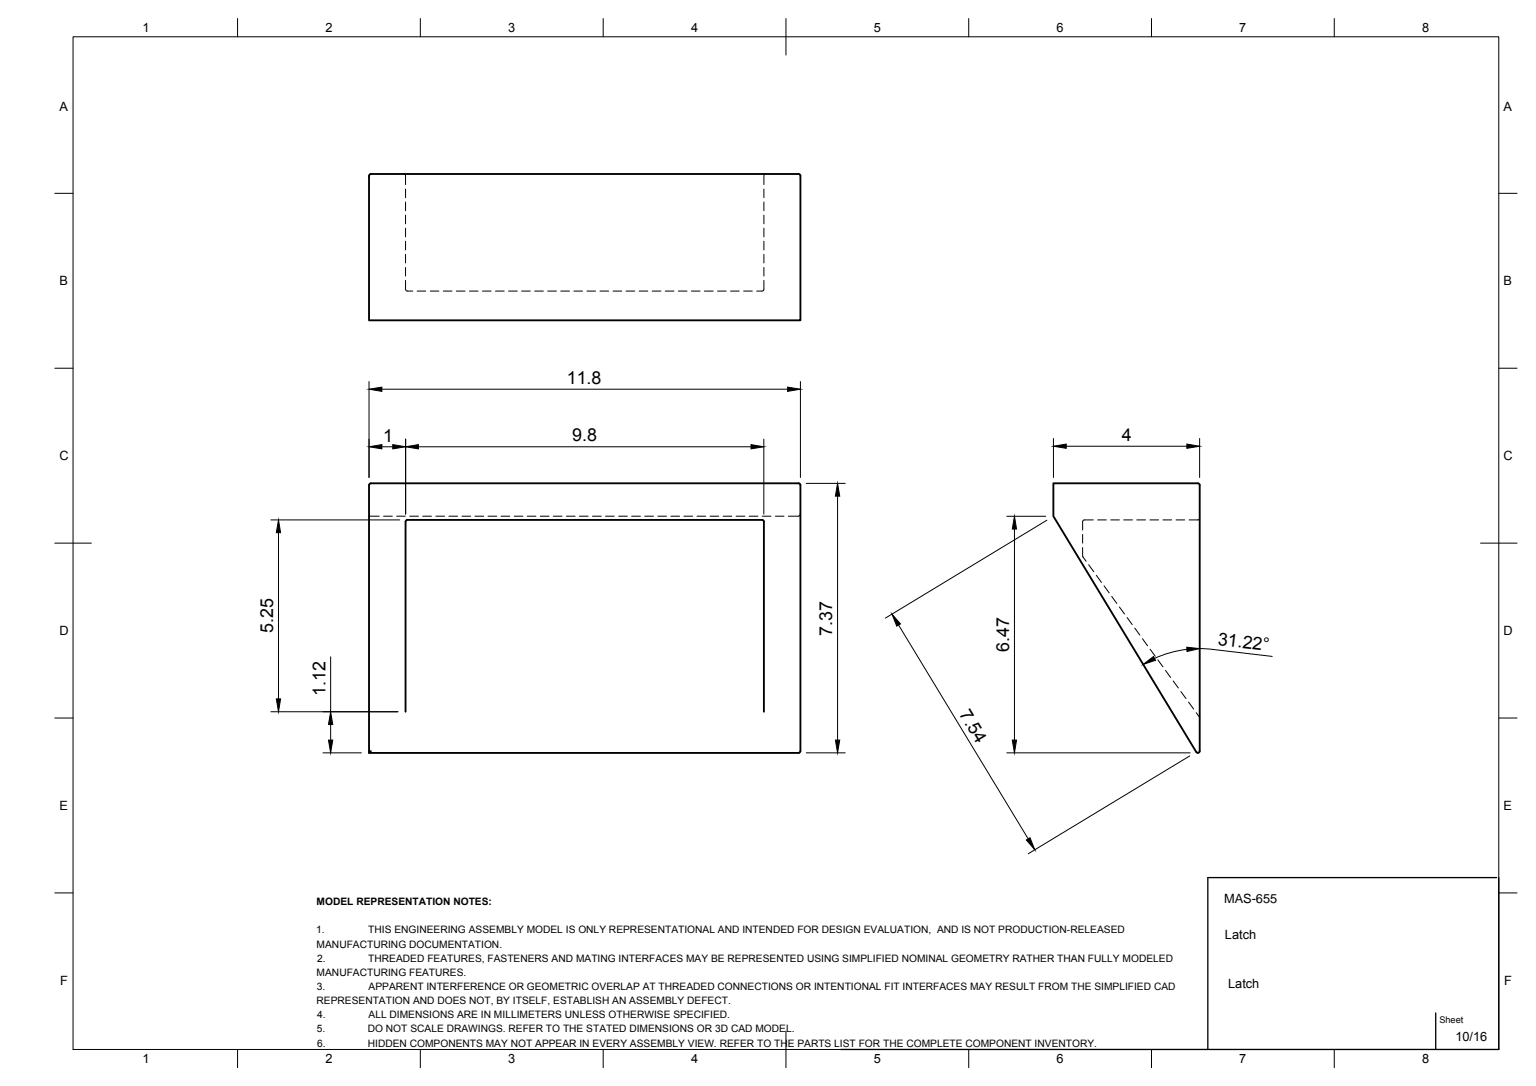
ISO-10303-21;
HEADER;
FILE_DESCRIPTION((''),'2;1');
FILE_NAME('Latch.step','2026-10-09T11:34:15-07:00',(''),(''),'','','');
FILE_SCHEMA (('AUTOMOTIVE_DESIGN { 1 0 10303 214 3 1 1 }'));
ENDSEC;
DATA;
#10=MECHANICAL_DESIGN_GEOMETRIC_PRESENTATION_REPRESENTATION('',(#642),#117170);
#389=ELLIPSE('',#52464,0.170018381359192,0.0999999999999989) ;
#390=ELLIPSE('',#52466,0.146308748884013,0.0499999999999989) ;
#391=ELLIPSE('',#52481,0.170018381359207,0.100000000000008) ;
#392=ELLIPSE('',#52483,0.146308748884017,0.0499999999999989) ;
#393=ELLIPSE('',#52506,0.0707106781186453,0.05) ;
#394=ELLIPSE('',#52515,0.0964689069078737,0.05) ;
#600=SHAPE_REPRESENTATION_RELATIONSHIP('SRR','None',#117255,#621) ;
#621=ADVANCED_BREP_SHAPE_REPRESENTATION('',(#663),#117163) ;
#642=STYLED_ITEM('',(#117355),#663) ;
#663=MANIFOLD_SOLID_BREP('Body1',#49071) ;
#737=FACE_BOUND('',#15539,.T.) ;
#2003=B_SPLINE_SURFACE_WITH_KNOTS('',3,3,((#88809,#88810,#88811,#88812,
#88813,#88814),(#88815,#88816,#88817,#88818,#88819,#88820),(#88821,#88822,
#88823,#88824,#88825,#88826),(#88827,#88828,#88829,#88830,#88831,#88832),
(#88833,#88834,#88835,#88836,#88837,#88838)),.UNSPECIFIED.,.F.,.F.,.F.,
(4,1,4),(4,1,1,4),(-0.00263861939634921,0.571428571428571,1.),(4.70975036097816,
5.38558740615393,5.83438635666676,6.28582392658612),.UNSPECIFIED.) ;
#2004=B_SPLINE_SURFACE_WITH_KNOTS('',3,3,((#88875,#88876,#88877,#88878,
#88879),(#88880,#88881,#88882,#88883,#88884),(#88885,#88886,#88887,#88888,
#88889),(#88890,#88891,#88892,#88893,#88894),(#88895,#88896,#88897,#88898,
#88899)),.UNSPECIFIED.,.F.,.F.,.F.,(4,1,4),(4,1,4),(-0.00515447126046521,
0.571428571428571,1.00290951547842),(-0.00515447124447774,0.673198425769152,
1.5759507980487),.UNSPECIFIED.) ;
#2204=SPHERICAL_SURFACE('',#52445,0.0499999999999989) ;
#2205=SPHERICAL_SURFACE('',#52449,0.0499999999999989) ;
#2206=SPHERICAL_SURFACE('',#52454,0.0499999999999901) ;
#2207=SPHERICAL_SURFACE('',#52470,0.0499999999999945) ;
#2208=SPHERICAL_SURFACE('',#52496,0.0499999999999989) ;
#2209=SPHERICAL_SURFACE('',#52500,0.0499999999999989) ;
#2210=SPHERICAL_SURFACE('',#52507,0.0499999999999989) ;
#2552=PLANE('',#52491) ;
#2553=PLANE('',#52492) ;
#2554=PLANE('',#52493) ;
#2555=PLANE('',#52494) ;
#2556=PLANE('',#52495) ;
#2557=PLANE('',#52520) ;
#2558=PLANE('',#52521) ;
#2559=PLANE('',#52522) ;
#2560=PLANE('',#52523) ;
#2561=PLANE('',#52524) ;
#2562=PLANE('',#52525) ;
#4549=LINE('',#88788,#7763) ;
#4550=LINE('',#88789,#7764) ;
#4551=LINE('',#88798,#7765) ;
#4552=LINE('',#88799,#7766) ;
#4553=LINE('',#88848,#7767) ;
#4554=LINE('',#88849,#7768) ;
#4555=LINE('',#88851,#7769) ;
#4556=LINE('',#88852,#7770) ;
#4557=LINE('',#88861,#7771) ;
#4558=LINE('',#88862,#7772) ;
#4559=LINE('',#88864,#7773) ;
#4560=LINE('',#88865,#7774) ;
#4561=LINE('',#88909,#7775) ;
#4562=LINE('',#88910,#7776) ;
#4563=LINE('',#88912,#7777) ;
#4564=LINE('',#88913,#7778) ;
#4565=LINE('',#88915,#7779) ;
#4566=LINE('',#88916,#7780) ;
#4567=LINE('',#88918,#7781) ;
#4568=LINE('',#88919,#7782) ;
#4569=LINE('',#88921,#7783) ;
#4570=LINE('',#88922,#7784) ;
#4571=LINE('',#88924,#7785) ;
#4572=LINE('',#88925,#7786) ;
#4573=LINE('',#88946,#7787) ;
#4574=LINE('',#88947,#7788) ;
#4575=LINE('',#88950,#7789) ;
#4576=LINE('',#88952,#7790) ;
#4577=LINE('',#88962,#7791) ;
#4578=LINE('',#88963,#7792) ;
#4579=LINE('',#88966,#7793) ;
#4580=LINE('',#88967,#7794) ;
#4581=LINE('',#88973,#7795) ;
#4582=LINE('',#88974,#7796) ;
#4583=LINE('',#88979,#7797) ;
#4584=LINE('',#88980,#7798) ;
#4585=LINE('',#88985,#7799) ;
#4586=LINE('',#88986,#7800) ;
#4587=LINE('',#88988,#7801) ;
#4588=LINE('',#88991,#7802) ;
#4589=LINE('',#88992,#7803) ;
#4590=LINE('',#88993,#7804) ;
#4591=LINE('',#88995,#7805) ;
#7763=VECTOR('',#62902,10.) ;
#7764=VECTOR('',#62903,10.) ;
#7765=VECTOR('',#62914,10.) ;
#7766=VECTOR('',#62915,10.) ;
#7767=VECTOR('',#62936,10.) ;
#7768=VECTOR('',#62937,10.) ;
#7769=VECTOR('',#62940,10.) ;
#7770=VECTOR('',#62941,10.) ;
#7771=VECTOR('',#62952,10.) ;
#7772=VECTOR('',#62953,10.) ;
#7773=VECTOR('',#62956,10.) ;
#7774=VECTOR('',#62957,10.) ;
#7775=VECTOR('',#62978,10.) ;
#7776=VECTOR('',#62979,10.) ;
#7777=VECTOR('',#62982,10.) ;
#7778=VECTOR('',#62983,10.) ;
#7779=VECTOR('',#62986,10.) ;
#7780=VECTOR('',#62987,10.) ;
#7781=VECTOR('',#62990,10.) ;
#7782=VECTOR('',#62991,10.) ;
#7783=VECTOR('',#62994,10.) ;
#7784=VECTOR('',#62995,10.) ;
#7785=VECTOR('',#62998,10.) ;
#7786=VECTOR('',#62999,10.) ;
#7787=VECTOR('',#63028,10.) ;
#7788=VECTOR('',#63029,10.) ;
#7789=VECTOR('',#63032,10.) ;
#7790=VECTOR('',#63033,10.) ;
#7791=VECTOR('',#63046,10.) ;
#7792=VECTOR('',#63047,10.) ;
#7793=VECTOR('',#63050,10.) ;
#7794=VECTOR('',#63051,10.) ;
#7795=VECTOR('',#63058,10.) ;
#7796=VECTOR('',#63059,10.) ;
#7797=VECTOR('',#63064,10.) ;
#7798=VECTOR('',#63065,10.) ;
#7799=VECTOR('',#63070,10.) ;
#7800=VECTOR('',#63071,10.) ;
#7801=VECTOR('',#63074,10.) ;
#7802=VECTOR('',#63077,10.) ;
#7803=VECTOR('',#63078,10.) ;
#7804=VECTOR('',#63079,10.) ;
#7805=VECTOR('',#63082,10.) ;
#10115=CYLINDRICAL_SURFACE('',#52453,0.05) ;
#10116=CYLINDRICAL_SURFACE('',#52458,0.05) ;
#10117=CYLINDRICAL_SURFACE('',#52468,0.05) ;
#10118=CYLINDRICAL_SURFACE('',#52469,0.05) ;
#10119=CYLINDRICAL_SURFACE('',#52474,0.05) ;
#10120=CYLINDRICAL_SURFACE('',#52475,0.05) ;
#10121=CYLINDRICAL_SURFACE('',#52485,0.05) ;
#10122=CYLINDRICAL_SURFACE('',#52486,0.05) ;
#10123=CYLINDRICAL_SURFACE('',#52487,0.05) ;
#10124=CYLINDRICAL_SURFACE('',#52488,0.05) ;
#10125=CYLINDRICAL_SURFACE('',#52489,0.05) ;
#10126=CYLINDRICAL_SURFACE('',#52490,0.05) ;
#10127=CYLINDRICAL_SURFACE('',#52504,0.05) ;
#10128=CYLINDRICAL_SURFACE('',#52505,0.05) ;
#10129=CYLINDRICAL_SURFACE('',#52511,0.05) ;
#10130=CYLINDRICAL_SURFACE('',#52512,0.05) ;
#10131=CYLINDRICAL_SURFACE('',#52514,0.05) ;
#10132=CYLINDRICAL_SURFACE('',#52516,0.05) ;
#10133=CYLINDRICAL_SURFACE('',#52518,0.05) ;
#12341=FACE_OUTER_BOUND('',#15500,.T.) ;
#12342=FACE_OUTER_BOUND('',#15501,.T.) ;
#12343=FACE_OUTER_BOUND('',#15502,.T.) ;
#12344=FACE_OUTER_BOUND('',#15503,.T.) ;
#12345=FACE_OUTER_BOUND('',#15504,.T.) ;
#12346=FACE_OUTER_BOUND('',#15505,.T.) ;
#12347=FACE_OUTER_BOUND('',#15506,.T.) ;
#12348=FACE_OUTER_BOUND('',#15507,.T.) ;
#12349=FACE_OUTER_BOUND('',#15508,.T.) ;
#12350=FACE_OUTER_BOUND('',#15509,.T.) ;
#12351=FACE_OUTER_BOUND('',#15510,.T.) ;
#12352=FACE_OUTER_BOUND('',#15511,.T.) ;
#12353=FACE_OUTER_BOUND('',#15512,.T.) ;
#12354=FACE_OUTER_BOUND('',#15513,.T.) ;
#12355=FACE_OUTER_BOUND('',#15514,.T.) ;
#12356=FACE_OUTER_BOUND('',#15515,.T.) ;
#12357=FACE_OUTER_BOUND('',#15516,.T.) ;
#12358=FACE_OUTER_BOUND('',#15517,.T.) ;
#12359=FACE_OUTER_BOUND('',#15518,.T.) ;
#12360=FACE_OUTER_BOUND('',#15519,.T.) ;
#12361=FACE_OUTER_BOUND('',#15520,.T.) ;
#12362=FACE_OUTER_BOUND('',#15521,.T.) ;
#12363=FACE_OUTER_BOUND('',#15522,.T.) ;
#12364=FACE_OUTER_BOUND('',#15523,.T.) ;
#12365=FACE_OUTER_BOUND('',#15524,.T.) ;
#12366=FACE_OUTER_BOUND('',#15525,.T.) ;
#12367=FACE_OUTER_BOUND('',#15526,.T.) ;
#12368=FACE_OUTER_BOUND('',#15527,.T.) ;
#12369=FACE_OUTER_BOUND('',#15528,.T.) ;
#12370=FACE_OUTER_BOUND('',#15529,.T.) ;
#12371=FACE_OUTER_BOUND('',#15530,.T.) ;
#12372=FACE_OUTER_BOUND('',#15531,.T.) ;
#12373=FACE_OUTER_BOUND('',#15532,.T.) ;
#12374=FACE_OUTER_BOUND('',#15533,.T.) ;
#12375=FACE_OUTER_BOUND('',#15534,.T.) ;
#12376=FACE_OUTER_BOUND('',#15535,.T.) ;
#12377=FACE_OUTER_BOUND('',#15536,.T.) ;
#12378=FACE_OUTER_BOUND('',#15537,.T.) ;
#12379=FACE_OUTER_BOUND('',#15538,.T.) ;
#12380=FACE_OUTER_BOUND('',#15540,.T.) ;
#12381=FACE_OUTER_BOUND('',#15541,.T.) ;
#15500=EDGE_LOOP('',(#38300,#38301,#38302)) ;
#15501=EDGE_LOOP('',(#38303,#38304,#38305)) ;
#15502=EDGE_LOOP('',(#38306,#38307,#38308,#38309)) ;
#15503=EDGE_LOOP('',(#38310,#38311,#38312)) ;
#15504=EDGE_LOOP('',(#38313,#38314,#38315,#38316)) ;
#15505=EDGE_LOOP('',(#38317,#38318,#38319,#38320)) ;
#15506=EDGE_LOOP('',(#38321,#38322,#38323,#38324)) ;
#15507=EDGE_LOOP('',(#38325,#38326,#38327,#38328)) ;
#15508=EDGE_LOOP('',(#38329,#38330,#38331,#38332)) ;
#15509=EDGE_LOOP('',(#38333,#38334,#38335)) ;
#15510=EDGE_LOOP('',(#38336,#38337,#38338,#38339)) ;
#15511=EDGE_LOOP('',(#38340,#38341,#38342,#38343)) ;
#15512=EDGE_LOOP('',(#38344,#38345,#38346,#38347)) ;
#15513=EDGE_LOOP('',(#38348,#38349,#38350,#38351)) ;
#15514=EDGE_LOOP('',(#38352,#38353,#38354,#38355)) ;
#15515=EDGE_LOOP('',(#38356,#38357,#38358,#38359)) ;
#15516=EDGE_LOOP('',(#38360,#38361,#38362,#38363)) ;
#15517=EDGE_LOOP('',(#38364,#38365,#38366,#38367)) ;
#15518=EDGE_LOOP('',(#38368,#38369,#38370,#38371)) ;
#15519=EDGE_LOOP('',(#38372,#38373,#38374,#38375)) ;
#15520=EDGE_LOOP('',(#38376,#38377,#38378,#38379)) ;
#15521=EDGE_LOOP('',(#38380,#38381,#38382,#38383)) ;
#15522=EDGE_LOOP('',(#38384,#38385,#38386,#38387)) ;
#15523=EDGE_LOOP('',(#38388,#38389,#38390,#38391)) ;
#15524=EDGE_LOOP('',(#38392,#38393,#38394,#38395)) ;
#15525=EDGE_LOOP('',(#38396,#38397,#38398)) ;
#15526=EDGE_LOOP('',(#38399,#38400,#38401)) ;
#15527=EDGE_LOOP('',(#38402,#38403,#38404,#38405)) ;
#15528=EDGE_LOOP('',(#38406,#38407,#38408,#38409)) ;
#15529=EDGE_LOOP('',(#38410,#38411,#38412)) ;
#15530=EDGE_LOOP('',(#38413,#38414,#38415,#38416)) ;
#15531=EDGE_LOOP('',(#38417,#38418,#38419,#38420,#38421)) ;
#15532=EDGE_LOOP('',(#38422,#38423,#38424,#38425)) ;
#15533=EDGE_LOOP('',(#38426,#38427,#38428,#38429)) ;
#15534=EDGE_LOOP('',(#38430,#38431,#38432,#38433)) ;
#15535=EDGE_LOOP('',(#38434,#38435,#38436,#38437)) ;
#15536=EDGE_LOOP('',(#38438,#38439,#38440,#38441,#38442,#38443,#38444)) ;
#15537=EDGE_LOOP('',(#38445,#38446,#38447,#38448)) ;
#15538=EDGE_LOOP('',(#38449,#38450,#38451,#38452)) ;
#15539=EDGE_LOOP('',(#38453,#38454,#38455,#38456,#38457,#38458,#38459,#38460)) ;
#15540=EDGE_LOOP('',(#38461,#38462,#38463,#38464,#38465)) ;
#15541=EDGE_LOOP('',(#38466,#38467,#38468,#38469)) ;
#18509=CIRCLE('',#52446,0.0499999999999901) ;
#18510=CIRCLE('',#52447,0.0499999999999989) ;
#18511=CIRCLE('',#52448,0.0499999999999989) ;
#18512=CIRCLE('',#52450,0.0499999999999989) ;
#18513=CIRCLE('',#52451,0.0499999999999989) ;
#18514=CIRCLE('',#52452,0.0500000000000149) ;
#18515=CIRCLE('',#52455,0.0499999999999989) ;
#18516=CIRCLE('',#52456,0.0499999999999901) ;
#18517=CIRCLE('',#52457,0.0499999999999945) ;
#18518=CIRCLE('',#52460,0.0499999999999989) ;
#18519=CIRCLE('',#52461,0.0500000000000034) ;
#18520=CIRCLE('',#52462,0.0999999999999979) ;
#18521=CIRCLE('',#52463,0.0499999999999901) ;
#18522=CIRCLE('',#52465,0.0499999999999989) ;
#18523=CIRCLE('',#52467,0.0499999999999989) ;
#18524=CIRCLE('',#52471,0.0500000000000005) ;
#18525=CIRCLE('',#52472,0.0499999999999945) ;
#18526=CIRCLE('',#52473,0.0499999999999989) ;
#18527=CIRCLE('',#52477,0.0999999999999801) ;
#18528=CIRCLE('',#52478,0.0499999999999989) ;
#18529=CIRCLE('',#52479,0.0499999999999901) ;
#18530=CIRCLE('',#52480,0.0500000000000034) ;
#18531=CIRCLE('',#52482,0.0500000000000077) ;
#18532=CIRCLE('',#52484,0.0500000000000034) ;
#18533=CIRCLE('',#52497,0.0499999999999989) ;
#18534=CIRCLE('',#52498,0.0499999999999989) ;
#18535=CIRCLE('',#52499,0.0499999999999901) ;
#18536=CIRCLE('',#52501,0.0499999999999901) ;
#18537=CIRCLE('',#52502,0.0499999999999989) ;
#18538=CIRCLE('',#52503,0.0499999999999989) ;
#18539=CIRCLE('',#52508,0.0499999999999989) ;
#18540=CIRCLE('',#52509,0.0499999999999989) ;
#18541=CIRCLE('',#52510,0.0500000000000243) ;
#18542=CIRCLE('',#52513,0.05) ;
#18543=CIRCLE('',#52517,0.05) ;
#18544=CIRCLE('',#52519,0.05) ;
#21669=VERTEX_POINT('',#88774) ;
#21670=VERTEX_POINT('',#88775) ;
#21671=VERTEX_POINT('',#88777) ;
#21672=VERTEX_POINT('',#88781) ;
#21673=VERTEX_POINT('',#88782) ;
#21674=VERTEX_POINT('',#88784) ;
#21675=VERTEX_POINT('',#88791) ;
#21676=VERTEX_POINT('',#88792) ;
#21677=VERTEX_POINT('',#88794) ;
#21678=VERTEX_POINT('',#88801) ;
#21679=VERTEX_POINT('',#88802) ;
#21680=VERTEX_POINT('',#88804) ;
#21681=VERTEX_POINT('',#88806) ;
#21682=VERTEX_POINT('',#88839) ;
#21683=VERTEX_POINT('',#88840) ;
#21684=VERTEX_POINT('',#88842) ;
#21685=VERTEX_POINT('',#88844) ;
#21686=VERTEX_POINT('',#88854) ;
#21687=VERTEX_POINT('',#88855) ;
#21688=VERTEX_POINT('',#88857) ;
#21689=VERTEX_POINT('',#88867) ;
#21690=VERTEX_POINT('',#88868) ;
#21691=VERTEX_POINT('',#88870) ;
#21692=VERTEX_POINT('',#88872) ;
#21693=VERTEX_POINT('',#88900) ;
#21694=VERTEX_POINT('',#88901) ;
#21695=VERTEX_POINT('',#88903) ;
#21696=VERTEX_POINT('',#88905) ;
#21697=VERTEX_POINT('',#88932) ;
#21698=VERTEX_POINT('',#88933) ;
#21699=VERTEX_POINT('',#88935) ;
#21700=VERTEX_POINT('',#88939) ;
#21701=VERTEX_POINT('',#88940) ;
#21702=VERTEX_POINT('',#88942) ;
#21703=VERTEX_POINT('',#88949) ;
#21704=VERTEX_POINT('',#88951) ;
#21705=VERTEX_POINT('',#88955) ;
#21706=VERTEX_POINT('',#88956) ;
#21707=VERTEX_POINT('',#88958) ;
#21708=VERTEX_POINT('',#88965) ;
#21709=VERTEX_POINT('',#88970) ;
#21710=VERTEX_POINT('',#88971) ;
#21711=VERTEX_POINT('',#88976) ;
#21712=VERTEX_POINT('',#88977) ;
#21713=VERTEX_POINT('',#88982) ;
#21714=VERTEX_POINT('',#88983) ;
#21715=VERTEX_POINT('',#88990) ;
#27428=EDGE_CURVE('',#21669,#21670,#18509,.F.) ;
#27429=EDGE_CURVE('',#21671,#21669,#18510,.F.) ;
#27430=EDGE_CURVE('',#21670,#21671,#18511,.F.) ;
#27431=EDGE_CURVE('',#21672,#21673,#18512,.F.) ;
#27432=EDGE_CURVE('',#21674,#21672,#18513,.F.) ;
#27433=EDGE_CURVE('',#21673,#21674,#18514,.F.) ;
#27434=EDGE_CURVE('',#21672,#21670,#4549,.T.) ;
#27435=EDGE_CURVE('',#21671,#21674,#4550,.T.) ;
#27436=EDGE_CURVE('',#21675,#21676,#18515,.F.) ;
#27437=EDGE_CURVE('',#21677,#21675,#18516,.F.) ;
#27438=EDGE_CURVE('',#21676,#21677,#18517,.F.) ;
#27439=EDGE_CURVE('',#21669,#21677,#4551,.T.) ;
#27440=EDGE_CURVE('',#21675,#21671,#4552,.T.) ;
#27441=EDGE_CURVE('',#21678,#21679,#18518,.F.) ;
#27442=EDGE_CURVE('',#21680,#21678,#18519,.T.) ;
#27443=EDGE_CURVE('',#21680,#21681,#18520,.T.) ;
#27444=EDGE_CURVE('',#21679,#21681,#18521,.T.) ;
#27445=EDGE_CURVE('',#21682,#21683,#389,.T.) ;
#27446=EDGE_CURVE('',#21684,#21683,#18522,.T.) ;
#27447=EDGE_CURVE('',#21685,#21684,#390,.F.) ;
#27448=EDGE_CURVE('',#21682,#21685,#18523,.T.) ;
#27449=EDGE_CURVE('',#21683,#21680,#4553,.T.) ;
#27450=EDGE_CURVE('',#21678,#21684,#4554,.T.) ;
#27451=EDGE_CURVE('',#21673,#21685,#4555,.T.) ;
#27452=EDGE_CURVE('',#21684,#21672,#4556,.T.) ;
#27453=EDGE_CURVE('',#21686,#21687,#18524,.F.) ;
#27454=EDGE_CURVE('',#21688,#21686,#18525,.F.) ;
#27455=EDGE_CURVE('',#21687,#21688,#18526,.F.) ;
#27456=EDGE_CURVE('',#21674,#21688,#4557,.T.) ;
#27457=EDGE_CURVE('',#21686,#21673,#4558,.T.) ;
#27458=EDGE_CURVE('',#21676,#21687,#4559,.T.) ;
#27459=EDGE_CURVE('',#21688,#21675,#4560,.T.) ;
#27460=EDGE_CURVE('',#21689,#21690,#18527,.T.) ;
#27461=EDGE_CURVE('',#21691,#21690,#18528,.T.) ;
#27462=EDGE_CURVE('',#21692,#21691,#18529,.F.) ;
#27463=EDGE_CURVE('',#21689,#21692,#18530,.T.) ;
#27464=EDGE_CURVE('',#21693,#21694,#391,.T.) ;
#27465=EDGE_CURVE('',#21695,#21694,#18531,.T.) ;
#27466=EDGE_CURVE('',#21696,#21695,#392,.F.) ;
#27467=EDGE_CURVE('',#21693,#21696,#18532,.T.) ;
#27468=EDGE_CURVE('',#21690,#21693,#4561,.T.) ;
#27469=EDGE_CURVE('',#21696,#21691,#4562,.T.) ;
#27470=EDGE_CURVE('',#21685,#21695,#4563,.T.) ;
#27471=EDGE_CURVE('',#21694,#21682,#4564,.T.) ;
#27472=EDGE_CURVE('',#21695,#21686,#4565,.T.) ;
#27473=EDGE_CURVE('',#21687,#21696,#4566,.T.) ;
#27474=EDGE_CURVE('',#21691,#21676,#4567,.T.) ;
#27475=EDGE_CURVE('',#21677,#21692,#4568,.T.) ;
#27476=EDGE_CURVE('',#21681,#21689,#4569,.T.) ;
#27477=EDGE_CURVE('',#21692,#21679,#4570,.T.) ;
#27478=EDGE_CURVE('',#21679,#21669,#4571,.T.) ;
#27479=EDGE_CURVE('',#21670,#21678,#4572,.T.) ;
#27480=EDGE_CURVE('',#21697,#21698,#18533,.F.) ;
#27481=EDGE_CURVE('',#21699,#21697,#18534,.F.) ;
#27482=EDGE_CURVE('',#21698,#21699,#18535,.F.) ;
#27483=EDGE_CURVE('',#21700,#21701,#18536,.F.) ;
#27484=EDGE_CURVE('',#21702,#21700,#18537,.F.) ;
#27485=EDGE_CURVE('',#21701,#21702,#18538,.F.) ;
#27486=EDGE_CURVE('',#21700,#21698,#4573,.T.) ;
#27487=EDGE_CURVE('',#21699,#21702,#4574,.T.) ;
#27488=EDGE_CURVE('',#21703,#21699,#4575,.T.) ;
#27489=EDGE_CURVE('',#21697,#21704,#4576,.T.) ;
#27490=EDGE_CURVE('',#21704,#21703,#393,.T.) ;
#27491=EDGE_CURVE('',#21705,#21706,#18539,.F.) ;
#27492=EDGE_CURVE('',#21707,#21705,#18540,.F.) ;
#27493=EDGE_CURVE('',#21706,#21707,#18541,.F.) ;
#27494=EDGE_CURVE('',#21705,#21701,#4577,.T.) ;
#27495=EDGE_CURVE('',#21702,#21707,#4578,.T.) ;
#27496=EDGE_CURVE('',#21708,#21706,#4579,.T.) ;
#27497=EDGE_CURVE('',#21707,#21703,#4580,.T.) ;
#27498=EDGE_CURVE('',#21704,#21708,#18542,.T.) ;
#27499=EDGE_CURVE('',#21709,#21710,#394,.T.) ;
#27500=EDGE_CURVE('',#21710,#21705,#4581,.T.) ;
#27501=EDGE_CURVE('',#21706,#21709,#4582,.T.) ;
#27502=EDGE_CURVE('',#21711,#21712,#18543,.T.) ;
#27503=EDGE_CURVE('',#21712,#21700,#4583,.T.) ;
#27504=EDGE_CURVE('',#21701,#21711,#4584,.T.) ;
#27505=EDGE_CURVE('',#21713,#21714,#18544,.T.) ;
#27506=EDGE_CURVE('',#21714,#21697,#4585,.T.) ;
#27507=EDGE_CURVE('',#21698,#21713,#4586,.T.) ;
#27508=EDGE_CURVE('',#21711,#21710,#4587,.T.) ;
#27509=EDGE_CURVE('',#21715,#21709,#4588,.T.) ;
#27510=EDGE_CURVE('',#21715,#21714,#4589,.T.) ;
#27511=EDGE_CURVE('',#21713,#21712,#4590,.T.) ;
#27512=EDGE_CURVE('',#21708,#21715,#4591,.T.) ;
#38300=ORIENTED_EDGE('',*,*,#27428,.F.) ;
#38301=ORIENTED_EDGE('',*,*,#27429,.F.) ;
#38302=ORIENTED_EDGE('',*,*,#27430,.F.) ;
#38303=ORIENTED_EDGE('',*,*,#27431,.F.) ;
#38304=ORIENTED_EDGE('',*,*,#27432,.F.) ;
#38305=ORIENTED_EDGE('',*,*,#27433,.F.) ;
#38306=ORIENTED_EDGE('',*,*,#27432,.T.) ;
#38307=ORIENTED_EDGE('',*,*,#27434,.T.) ;
#38308=ORIENTED_EDGE('',*,*,#27430,.T.) ;
#38309=ORIENTED_EDGE('',*,*,#27435,.T.) ;
#38310=ORIENTED_EDGE('',*,*,#27436,.F.) ;
#38311=ORIENTED_EDGE('',*,*,#27437,.F.) ;
#38312=ORIENTED_EDGE('',*,*,#27438,.F.) ;
#38313=ORIENTED_EDGE('',*,*,#27429,.T.) ;
#38314=ORIENTED_EDGE('',*,*,#27439,.T.) ;
#38315=ORIENTED_EDGE('',*,*,#27437,.T.) ;
#38316=ORIENTED_EDGE('',*,*,#27440,.T.) ;
#38317=ORIENTED_EDGE('',*,*,#27441,.F.) ;
#38318=ORIENTED_EDGE('',*,*,#27442,.F.) ;
#38319=ORIENTED_EDGE('',*,*,#27443,.T.) ;
#38320=ORIENTED_EDGE('',*,*,#27444,.F.) ;
#38321=ORIENTED_EDGE('',*,*,#27445,.T.) ;
#38322=ORIENTED_EDGE('',*,*,#27446,.F.) ;
#38323=ORIENTED_EDGE('',*,*,#27447,.F.) ;
#38324=ORIENTED_EDGE('',*,*,#27448,.F.) ;
#38325=ORIENTED_EDGE('',*,*,#27446,.T.) ;
#38326=ORIENTED_EDGE('',*,*,#27449,.T.) ;
#38327=ORIENTED_EDGE('',*,*,#27442,.T.) ;
#38328=ORIENTED_EDGE('',*,*,#27450,.T.) ;
#38329=ORIENTED_EDGE('',*,*,#27431,.T.) ;
#38330=ORIENTED_EDGE('',*,*,#27451,.T.) ;
#38331=ORIENTED_EDGE('',*,*,#27447,.T.) ;
#38332=ORIENTED_EDGE('',*,*,#27452,.T.) ;
#38333=ORIENTED_EDGE('',*,*,#27453,.F.) ;
#38334=ORIENTED_EDGE('',*,*,#27454,.F.) ;
#38335=ORIENTED_EDGE('',*,*,#27455,.F.) ;
#38336=ORIENTED_EDGE('',*,*,#27433,.T.) ;
#38337=ORIENTED_EDGE('',*,*,#27456,.T.) ;
#38338=ORIENTED_EDGE('',*,*,#27454,.T.) ;
#38339=ORIENTED_EDGE('',*,*,#27457,.T.) ;
#38340=ORIENTED_EDGE('',*,*,#27436,.T.) ;
#38341=ORIENTED_EDGE('',*,*,#27458,.T.) ;
#38342=ORIENTED_EDGE('',*,*,#27455,.T.) ;
#38343=ORIENTED_EDGE('',*,*,#27459,.T.) ;
#38344=ORIENTED_EDGE('',*,*,#27460,.T.) ;
#38345=ORIENTED_EDGE('',*,*,#27461,.F.) ;
#38346=ORIENTED_EDGE('',*,*,#27462,.F.) ;
#38347=ORIENTED_EDGE('',*,*,#27463,.F.) ;
#38348=ORIENTED_EDGE('',*,*,#27464,.T.) ;
#38349=ORIENTED_EDGE('',*,*,#27465,.F.) ;
#38350=ORIENTED_EDGE('',*,*,#27466,.F.) ;
#38351=ORIENTED_EDGE('',*,*,#27467,.F.) ;
#38352=ORIENTED_EDGE('',*,*,#27461,.T.) ;
#38353=ORIENTED_EDGE('',*,*,#27468,.T.) ;
#38354=ORIENTED_EDGE('',*,*,#27467,.T.) ;
#38355=ORIENTED_EDGE('',*,*,#27469,.T.) ;
#38356=ORIENTED_EDGE('',*,*,#27448,.T.) ;
#38357=ORIENTED_EDGE('',*,*,#27470,.T.) ;
#38358=ORIENTED_EDGE('',*,*,#27465,.T.) ;
#38359=ORIENTED_EDGE('',*,*,#27471,.T.) ;
#38360=ORIENTED_EDGE('',*,*,#27466,.T.) ;
#38361=ORIENTED_EDGE('',*,*,#27472,.T.) ;
#38362=ORIENTED_EDGE('',*,*,#27453,.T.) ;
#38363=ORIENTED_EDGE('',*,*,#27473,.T.) ;
#38364=ORIENTED_EDGE('',*,*,#27462,.T.) ;
#38365=ORIENTED_EDGE('',*,*,#27474,.T.) ;
#38366=ORIENTED_EDGE('',*,*,#27438,.T.) ;
#38367=ORIENTED_EDGE('',*,*,#27475,.T.) ;
#38368=ORIENTED_EDGE('',*,*,#27444,.T.) ;
#38369=ORIENTED_EDGE('',*,*,#27476,.T.) ;
#38370=ORIENTED_EDGE('',*,*,#27463,.T.) ;
#38371=ORIENTED_EDGE('',*,*,#27477,.T.) ;
#38372=ORIENTED_EDGE('',*,*,#27441,.T.) ;
#38373=ORIENTED_EDGE('',*,*,#27478,.T.) ;
#38374=ORIENTED_EDGE('',*,*,#27428,.T.) ;
#38375=ORIENTED_EDGE('',*,*,#27479,.T.) ;
#38376=ORIENTED_EDGE('',*,*,#27435,.F.) ;
#38377=ORIENTED_EDGE('',*,*,#27440,.F.) ;
#38378=ORIENTED_EDGE('',*,*,#27459,.F.) ;
#38379=ORIENTED_EDGE('',*,*,#27456,.F.) ;
#38380=ORIENTED_EDGE('',*,*,#27439,.F.) ;
#38381=ORIENTED_EDGE('',*,*,#27478,.F.) ;
#38382=ORIENTED_EDGE('',*,*,#27477,.F.) ;
#38383=ORIENTED_EDGE('',*,*,#27475,.F.) ;
#38384=ORIENTED_EDGE('',*,*,#27450,.F.) ;
#38385=ORIENTED_EDGE('',*,*,#27479,.F.) ;
#38386=ORIENTED_EDGE('',*,*,#27434,.F.) ;
#38387=ORIENTED_EDGE('',*,*,#27452,.F.) ;
#38388=ORIENTED_EDGE('',*,*,#27451,.F.) ;
#38389=ORIENTED_EDGE('',*,*,#27457,.F.) ;
#38390=ORIENTED_EDGE('',*,*,#27472,.F.) ;
#38391=ORIENTED_EDGE('',*,*,#27470,.F.) ;
#38392=ORIENTED_EDGE('',*,*,#27469,.F.) ;
#38393=ORIENTED_EDGE('',*,*,#27473,.F.) ;
#38394=ORIENTED_EDGE('',*,*,#27458,.F.) ;
#38395=ORIENTED_EDGE('',*,*,#27474,.F.) ;
#38396=ORIENTED_EDGE('',*,*,#27480,.F.) ;
#38397=ORIENTED_EDGE('',*,*,#27481,.F.) ;
#38398=ORIENTED_EDGE('',*,*,#27482,.F.) ;
#38399=ORIENTED_EDGE('',*,*,#27483,.F.) ;
#38400=ORIENTED_EDGE('',*,*,#27484,.F.) ;
#38401=ORIENTED_EDGE('',*,*,#27485,.F.) ;
#38402=ORIENTED_EDGE('',*,*,#27484,.T.) ;
#38403=ORIENTED_EDGE('',*,*,#27486,.T.) ;
#38404=ORIENTED_EDGE('',*,*,#27482,.T.) ;
#38405=ORIENTED_EDGE('',*,*,#27487,.T.) ;
#38406=ORIENTED_EDGE('',*,*,#27488,.T.) ;
#38407=ORIENTED_EDGE('',*,*,#27481,.T.) ;
#38408=ORIENTED_EDGE('',*,*,#27489,.T.) ;
#38409=ORIENTED_EDGE('',*,*,#27490,.T.) ;
#38410=ORIENTED_EDGE('',*,*,#27491,.F.) ;
#38411=ORIENTED_EDGE('',*,*,#27492,.F.) ;
#38412=ORIENTED_EDGE('',*,*,#27493,.F.) ;
#38413=ORIENTED_EDGE('',*,*,#27492,.T.) ;
#38414=ORIENTED_EDGE('',*,*,#27494,.T.) ;
#38415=ORIENTED_EDGE('',*,*,#27485,.T.) ;
#38416=ORIENTED_EDGE('',*,*,#27495,.T.) ;
#38417=ORIENTED_EDGE('',*,*,#27496,.T.) ;
#38418=ORIENTED_EDGE('',*,*,#27493,.T.) ;
#38419=ORIENTED_EDGE('',*,*,#27497,.T.) ;
#38420=ORIENTED_EDGE('',*,*,#27490,.F.) ;
#38421=ORIENTED_EDGE('',*,*,#27498,.T.) ;
#38422=ORIENTED_EDGE('',*,*,#27499,.T.) ;
#38423=ORIENTED_EDGE('',*,*,#27500,.T.) ;
#38424=ORIENTED_EDGE('',*,*,#27491,.T.) ;
#38425=ORIENTED_EDGE('',*,*,#27501,.T.) ;
#38426=ORIENTED_EDGE('',*,*,#27502,.T.) ;
#38427=ORIENTED_EDGE('',*,*,#27503,.T.) ;
#38428=ORIENTED_EDGE('',*,*,#27483,.T.) ;
#38429=ORIENTED_EDGE('',*,*,#27504,.T.) ;
#38430=ORIENTED_EDGE('',*,*,#27505,.T.) ;
#38431=ORIENTED_EDGE('',*,*,#27506,.T.) ;
#38432=ORIENTED_EDGE('',*,*,#27480,.T.) ;
#38433=ORIENTED_EDGE('',*,*,#27507,.T.) ;
#38434=ORIENTED_EDGE('',*,*,#27504,.F.) ;
#38435=ORIENTED_EDGE('',*,*,#27494,.F.) ;
#38436=ORIENTED_EDGE('',*,*,#27500,.F.) ;
#38437=ORIENTED_EDGE('',*,*,#27508,.F.) ;
#38438=ORIENTED_EDGE('',*,*,#27502,.F.) ;
#38439=ORIENTED_EDGE('',*,*,#27508,.T.) ;
#38440=ORIENTED_EDGE('',*,*,#27499,.F.) ;
#38441=ORIENTED_EDGE('',*,*,#27509,.F.) ;
#38442=ORIENTED_EDGE('',*,*,#27510,.T.) ;
#38443=ORIENTED_EDGE('',*,*,#27505,.F.) ;
#38444=ORIENTED_EDGE('',*,*,#27511,.T.) ;
#38445=ORIENTED_EDGE('',*,*,#27501,.F.) ;
#38446=ORIENTED_EDGE('',*,*,#27496,.F.) ;
#38447=ORIENTED_EDGE('',*,*,#27512,.T.) ;
#38448=ORIENTED_EDGE('',*,*,#27509,.T.) ;
#38449=ORIENTED_EDGE('',*,*,#27487,.F.) ;
#38450=ORIENTED_EDGE('',*,*,#27488,.F.) ;
#38451=ORIENTED_EDGE('',*,*,#27497,.F.) ;
#38452=ORIENTED_EDGE('',*,*,#27495,.F.) ;
#38453=ORIENTED_EDGE('',*,*,#27445,.F.) ;
#38454=ORIENTED_EDGE('',*,*,#27471,.F.) ;
#38455=ORIENTED_EDGE('',*,*,#27464,.F.) ;
#38456=ORIENTED_EDGE('',*,*,#27468,.F.) ;
#38457=ORIENTED_EDGE('',*,*,#27460,.F.) ;
#38458=ORIENTED_EDGE('',*,*,#27476,.F.) ;
#38459=ORIENTED_EDGE('',*,*,#27443,.F.) ;
#38460=ORIENTED_EDGE('',*,*,#27449,.F.) ;
#38461=ORIENTED_EDGE('',*,*,#27506,.F.) ;
#38462=ORIENTED_EDGE('',*,*,#27510,.F.) ;
#38463=ORIENTED_EDGE('',*,*,#27512,.F.) ;
#38464=ORIENTED_EDGE('',*,*,#27498,.F.) ;
#38465=ORIENTED_EDGE('',*,*,#27489,.F.) ;
#38466=ORIENTED_EDGE('',*,*,#27503,.F.) ;
#38467=ORIENTED_EDGE('',*,*,#27511,.F.) ;
#38468=ORIENTED_EDGE('',*,*,#27507,.F.) ;
#38469=ORIENTED_EDGE('',*,*,#27486,.F.) ;
#45713=TOROIDAL_SURFACE('',#52459,0.0999999999999801,0.0499999999999901) ;
#45714=TOROIDAL_SURFACE('',#52476,0.0999999999999801,0.0500000000000034) ;
#47559=ADVANCED_FACE('',(#12341),#2204,.F.) ;
#47560=ADVANCED_FACE('',(#12342),#2205,.F.) ;
#47561=ADVANCED_FACE('',(#12343),#10115,.F.) ;
#47562=ADVANCED_FACE('',(#12344),#2206,.F.) ;
#47563=ADVANCED_FACE('',(#12345),#10116,.F.) ;
#47564=ADVANCED_FACE('',(#12346),#45713,.T.) ;
#47565=ADVANCED_FACE('',(#12347),#2003,.F.) ;
#47566=ADVANCED_FACE('',(#12348),#10117,.T.) ;
#47567=ADVANCED_FACE('',(#12349),#10118,.F.) ;
#47568=ADVANCED_FACE('',(#12350),#2207,.F.) ;
#47569=ADVANCED_FACE('',(#12351),#10119,.F.) ;
#47570=ADVANCED_FACE('',(#12352),#10120,.F.) ;
#47571=ADVANCED_FACE('',(#12353),#45714,.T.) ;
#47572=ADVANCED_FACE('',(#12354),#2004,.F.) ;
#47573=ADVANCED_FACE('',(#12355),#10121,.T.) ;
#47574=ADVANCED_FACE('',(#12356),#10122,.T.) ;
#47575=ADVANCED_FACE('',(#12357),#10123,.F.) ;
#47576=ADVANCED_FACE('',(#12358),#10124,.F.) ;
#47577=ADVANCED_FACE('',(#12359),#10125,.T.) ;
#47578=ADVANCED_FACE('',(#12360),#10126,.F.) ;
#47579=ADVANCED_FACE('',(#12361),#2552,.F.) ;
#47580=ADVANCED_FACE('',(#12362),#2553,.F.) ;
#47581=ADVANCED_FACE('',(#12363),#2554,.F.) ;
#47582=ADVANCED_FACE('',(#12364),#2555,.T.) ;
#47583=ADVANCED_FACE('',(#12365),#2556,.F.) ;
#47584=ADVANCED_FACE('',(#12366),#2208,.T.) ;
#47585=ADVANCED_FACE('',(#12367),#2209,.T.) ;
#47586=ADVANCED_FACE('',(#12368),#10127,.T.) ;
#47587=ADVANCED_FACE('',(#12369),#10128,.T.) ;
#47588=ADVANCED_FACE('',(#12370),#2210,.T.) ;
#47589=ADVANCED_FACE('',(#12371),#10129,.T.) ;
#47590=ADVANCED_FACE('',(#12372),#10130,.T.) ;
#47591=ADVANCED_FACE('',(#12373),#10131,.T.) ;
#47592=ADVANCED_FACE('',(#12374),#10132,.T.) ;
#47593=ADVANCED_FACE('',(#12375),#10133,.T.) ;
#47594=ADVANCED_FACE('',(#12376),#2557,.T.) ;
#47595=ADVANCED_FACE('',(#12377),#2558,.T.) ;
#47596=ADVANCED_FACE('',(#12378),#2559,.T.) ;
#47597=ADVANCED_FACE('',(#12379,#737),#2560,.F.) ;
#47598=ADVANCED_FACE('',(#12380),#2561,.T.) ;
#47599=ADVANCED_FACE('',(#12381),#2562,.T.) ;
#49071=CLOSED_SHELL('',(#47559,#47560,#47561,#47562,#47563,#47564,#47565,
#47566,#47567,#47568,#47569,#47570,#47571,#47572,#47573,#47574,#47575,#47576,
#47577,#47578,#47579,#47580,#47581,#47582,#47583,#47584,#47585,#47586,#47587,
#47588,#47589,#47590,#47591,#47592,#47593,#47594,#47595,#47596,#47597,#47598,
#47599)) ;
#52444=AXIS2_PLACEMENT_3D('',#88772,#62882,#62883) ;
#52445=AXIS2_PLACEMENT_3D('',#88773,#62884,#62885) ;
#52446=AXIS2_PLACEMENT_3D('',#88776,#62886,#62887) ;
#52447=AXIS2_PLACEMENT_3D('',#88778,#62888,#62889) ;
#52448=AXIS2_PLACEMENT_3D('',#88779,#62890,#62891) ;
#52449=AXIS2_PLACEMENT_3D('',#88780,#62892,#62893) ;
#52450=AXIS2_PLACEMENT_3D('',#88783,#62894,#62895) ;
#52451=AXIS2_PLACEMENT_3D('',#88785,#62896,#62897) ;
#52452=AXIS2_PLACEMENT_3D('',#88786,#62898,#62899) ;
#52453=AXIS2_PLACEMENT_3D('',#88787,#62900,#62901) ;
#52454=AXIS2_PLACEMENT_3D('',#88790,#62904,#62905) ;
#52455=AXIS2_PLACEMENT_3D('',#88793,#62906,#62907) ;
#52456=AXIS2_PLACEMENT_3D('',#88795,#62908,#62909) ;
#52457=AXIS2_PLACEMENT_3D('',#88796,#62910,#62911) ;
#52458=AXIS2_PLACEMENT_3D('',#88797,#62912,#62913) ;
#52459=AXIS2_PLACEMENT_3D('',#88800,#62916,#62917) ;
#52460=AXIS2_PLACEMENT_3D('',#88803,#62918,#62919) ;
#52461=AXIS2_PLACEMENT_3D('',#88805,#62920,#62921) ;
#52462=AXIS2_PLACEMENT_3D('',#88807,#62922,#62923) ;
#52463=AXIS2_PLACEMENT_3D('',#88808,#62924,#62925) ;
#52464=AXIS2_PLACEMENT_3D('',#88841,#62926,#62927) ;
#52465=AXIS2_PLACEMENT_3D('',#88843,#62928,#62929) ;
#52466=AXIS2_PLACEMENT_3D('',#88845,#62930,#62931) ;
#52467=AXIS2_PLACEMENT_3D('',#88846,#62932,#62933) ;
#52468=AXIS2_PLACEMENT_3D('',#88847,#62934,#62935) ;
#52469=AXIS2_PLACEMENT_3D('',#88850,#62938,#62939) ;
#52470=AXIS2_PLACEMENT_3D('',#88853,#62942,#62943) ;
#52471=AXIS2_PLACEMENT_3D('',#88856,#62944,#62945) ;
#52472=AXIS2_PLACEMENT_3D('',#88858,#62946,#62947) ;
#52473=AXIS2_PLACEMENT_3D('',#88859,#62948,#62949) ;
#52474=AXIS2_PLACEMENT_3D('',#88860,#62950,#62951) ;
#52475=AXIS2_PLACEMENT_3D('',#88863,#62954,#62955) ;
#52476=AXIS2_PLACEMENT_3D('',#88866,#62958,#62959) ;
#52477=AXIS2_PLACEMENT_3D('',#88869,#62960,#62961) ;
#52478=AXIS2_PLACEMENT_3D('',#88871,#62962,#62963) ;
#52479=AXIS2_PLACEMENT_3D('',#88873,#62964,#62965) ;
#52480=AXIS2_PLACEMENT_3D('',#88874,#62966,#62967) ;
#52481=AXIS2_PLACEMENT_3D('',#88902,#62968,#62969) ;
#52482=AXIS2_PLACEMENT_3D('',#88904,#62970,#62971) ;
#52483=AXIS2_PLACEMENT_3D('',#88906,#62972,#62973) ;
#52484=AXIS2_PLACEMENT_3D('',#88907,#62974,#62975) ;
#52485=AXIS2_PLACEMENT_3D('',#88908,#62976,#62977) ;
#52486=AXIS2_PLACEMENT_3D('',#88911,#62980,#62981) ;
#52487=AXIS2_PLACEMENT_3D('',#88914,#62984,#62985) ;
#52488=AXIS2_PLACEMENT_3D('',#88917,#62988,#62989) ;
#52489=AXIS2_PLACEMENT_3D('',#88920,#62992,#62993) ;
#52490=AXIS2_PLACEMENT_3D('',#88923,#62996,#62997) ;
#52491=AXIS2_PLACEMENT_3D('',#88926,#63000,#63001) ;
#52492=AXIS2_PLACEMENT_3D('',#88927,#63002,#63003) ;
#52493=AXIS2_PLACEMENT_3D('',#88928,#63004,#63005) ;
#52494=AXIS2_PLACEMENT_3D('',#88929,#63006,#63007) ;
#52495=AXIS2_PLACEMENT_3D('',#88930,#63008,#63009) ;
#52496=AXIS2_PLACEMENT_3D('',#88931,#63010,#63011) ;
#52497=AXIS2_PLACEMENT_3D('',#88934,#63012,#63013) ;
#52498=AXIS2_PLACEMENT_3D('',#88936,#63014,#63015) ;
#52499=AXIS2_PLACEMENT_3D('',#88937,#63016,#63017) ;
#52500=AXIS2_PLACEMENT_3D('',#88938,#63018,#63019) ;
#52501=AXIS2_PLACEMENT_3D('',#88941,#63020,#63021) ;
#52502=AXIS2_PLACEMENT_3D('',#88943,#63022,#63023) ;
#52503=AXIS2_PLACEMENT_3D('',#88944,#63024,#63025) ;
#52504=AXIS2_PLACEMENT_3D('',#88945,#63026,#63027) ;
#52505=AXIS2_PLACEMENT_3D('',#88948,#63030,#63031) ;
#52506=AXIS2_PLACEMENT_3D('',#88953,#63034,#63035) ;
#52507=AXIS2_PLACEMENT_3D('',#88954,#63036,#63037) ;
#52508=AXIS2_PLACEMENT_3D('',#88957,#63038,#63039) ;
#52509=AXIS2_PLACEMENT_3D('',#88959,#63040,#63041) ;
#52510=AXIS2_PLACEMENT_3D('',#88960,#63042,#63043) ;
#52511=AXIS2_PLACEMENT_3D('',#88961,#63044,#63045) ;
#52512=AXIS2_PLACEMENT_3D('',#88964,#63048,#63049) ;
#52513=AXIS2_PLACEMENT_3D('',#88968,#63052,#63053) ;
#52514=AXIS2_PLACEMENT_3D('',#88969,#63054,#63055) ;
#52515=AXIS2_PLACEMENT_3D('',#88972,#63056,#63057) ;
#52516=AXIS2_PLACEMENT_3D('',#88975,#63060,#63061) ;
#52517=AXIS2_PLACEMENT_3D('',#88978,#63062,#63063) ;
#52518=AXIS2_PLACEMENT_3D('',#88981,#63066,#63067) ;
#52519=AXIS2_PLACEMENT_3D('',#88984,#63068,#63069) ;
#52520=AXIS2_PLACEMENT_3D('',#88987,#63072,#63073) ;
#52521=AXIS2_PLACEMENT_3D('',#88989,#63075,#63076) ;
#52522=AXIS2_PLACEMENT_3D('',#88994,#63080,#63081) ;
#52523=AXIS2_PLACEMENT_3D('',#88996,#63083,#63084) ;
#52524=AXIS2_PLACEMENT_3D('',#88997,#63085,#63086) ;
#52525=AXIS2_PLACEMENT_3D('',#88998,#63087,#63088) ;
#62882=DIRECTION('axis',(0.,0.,1.)) ;
#62883=DIRECTION('refdir',(1.,0.,0.)) ;
#62884=DIRECTION('center_axis',(0.408248290463875,-0.81649658092775,-0.408248290463804)) ;
#62885=DIRECTION('ref_axis',(0.577350269189578,0.577350269189721,-0.577350269189578)) ;
#62886=DIRECTION('center_axis',(0.,0.,1.)) ;
#62887=DIRECTION('ref_axis',(0.,1.,0.)) ;
#62888=DIRECTION('center_axis',(-1.,0.,0.)) ;
#62889=DIRECTION('ref_axis',(0.,0.,-1.)) ;
#62890=DIRECTION('center_axis',(0.,-1.,0.)) ;
#62891=DIRECTION('ref_axis',(1.,0.,0.)) ;
#62892=DIRECTION('center_axis',(-0.132437337493908,-0.961810237044439,0.239544191234197)) ;
#62893=DIRECTION('ref_axis',(0.465369435981278,-0.273717131207721,-0.841730491391326)) ;
#62894=DIRECTION('center_axis',(0.,-0.808736084303588,0.588171697674497)) ;
#62895=DIRECTION('ref_axis',(1.,0.,0.)) ;
#62896=DIRECTION('center_axis',(7.10542735760115E-13,1.,0.)) ;
#62897=DIRECTION('ref_axis',(0.,0.,-1.)) ;
#62898=DIRECTION('center_axis',(-1.,0.,0.)) ;
#62899=DIRECTION('ref_axis',(0.,-0.588171697675046,-0.808736084303189)) ;
#62900=DIRECTION('center_axis',(1.41426179436738E-51,-1.,-5.60383084497445E-34)) ;
#62901=DIRECTION('ref_axis',(0.707106781186485,3.96250679110413E-34,-0.70710678118661)) ;
#62902=DIRECTION('',(-1.41426179436738E-51,1.,5.60383084497445E-34)) ;
#62903=DIRECTION('',(1.41426179436738E-51,-1.,-5.60383084497445E-34)) ;
#62904=DIRECTION('center_axis',(-0.408248290463768,-0.816496580927821,-0.408248290463768)) ;
#62905=DIRECTION('ref_axis',(-0.577350269189673,0.577350269189389,-0.577350269189815)) ;
#62906=DIRECTION('center_axis',(0.,-1.,0.)) ;
#62907=DIRECTION('ref_axis',(0.,0.,-1.)) ;
#62908=DIRECTION('center_axis',(1.,0.,8.88178419700144E-14)) ;
#62909=DIRECTION('ref_axis',(0.,1.,0.)) ;
#62910=DIRECTION('center_axis',(0.,0.,1.)) ;
#62911=DIRECTION('ref_axis',(-1.,0.,0.)) ;
#62912=DIRECTION('center_axis',(1.,0.,2.52374105052742E-18)) ;
#62913=DIRECTION('ref_axis',(1.78455441078759E-18,0.707106781186234,-0.707106781186862)) ;
#62914=DIRECTION('',(-1.,0.,-2.52374105052742E-18)) ;
#62915=DIRECTION('',(1.,0.,2.52374105052742E-18)) ;
#62916=DIRECTION('center_axis',(0.,0.,-1.)) ;
#62917=DIRECTION('ref_axis',(-1.,0.,0.)) ;
#62918=DIRECTION('center_axis',(0.,0.,-1.)) ;
#62919=DIRECTION('ref_axis',(1.,0.,0.)) ;
#62920=DIRECTION('center_axis',(0.,-1.,0.)) ;
#62921=DIRECTION('ref_axis',(0.,0.,1.)) ;
#62922=DIRECTION('center_axis',(-2.52374105052742E-18,-5.60383084497445E-34,
1.)) ;
#62923=DIRECTION('ref_axis',(0.70710678118661,0.707106781186485,1.78455441078696E-18)) ;
#62924=DIRECTION('center_axis',(-1.,0.,0.)) ;
#62925=DIRECTION('ref_axis',(0.,-1.,0.)) ;
#62926=DIRECTION('center_axis',(-2.52374105052742E-18,-5.60383084497445E-34,
1.)) ;
#62927=DIRECTION('ref_axis',(-5.10157625931022E-17,-1.,-6.89133658777618E-34)) ;
#62928=DIRECTION('center_axis',(0.,1.,0.)) ;
#62929=DIRECTION('ref_axis',(-1.,0.,0.)) ;
#62930=DIRECTION('center_axis',(0.,-0.276379946678477,-0.961048450950316)) ;
#62931=DIRECTION('ref_axis',(0.,-0.961048450950316,0.276379946678477)) ;
#62932=DIRECTION('center_axis',(-1.,0.,0.)) ;
#62933=DIRECTION('ref_axis',(0.,0.,1.)) ;
#62934=DIRECTION('center_axis',(1.41426179436738E-51,-1.,-5.60383084497445E-34)) ;
#62935=DIRECTION('ref_axis',(-0.707106781186422,-3.96250679110448E-34,0.707106781186673)) ;
#62936=DIRECTION('',(-1.41426179436738E-51,1.,5.60383084497445E-34)) ;
#62937=DIRECTION('',(1.41426179436738E-51,-1.,-5.60383084497445E-34)) ;
#62938=DIRECTION('center_axis',(-1.14376454575628E-51,0.80873608430319,
-0.588171697675045)) ;
#62939=DIRECTION('ref_axis',(0.707106781186249,-0.415900195928203,-0.571862769401282)) ;
#62940=DIRECTION('',(1.14376454575628E-51,-0.80873608430319,0.588171697675045)) ;
#62941=DIRECTION('',(-1.14376454575628E-51,0.80873608430319,-0.588171697675045)) ;
#62942=DIRECTION('center_axis',(0.132437337493908,-0.961810237044439,0.239544191234197)) ;
#62943=DIRECTION('ref_axis',(-0.465369435981306,-0.273717131207737,-0.841730491391305)) ;
#62944=DIRECTION('center_axis',(8.88082395220738E-13,-0.808736084303066,
0.588171697675215)) ;
#62945=DIRECTION('ref_axis',(1.19592671626956E-29,-0.588171697675215,-0.808736084303066)) ;
#62946=DIRECTION('center_axis',(1.,0.,0.)) ;
#62947=DIRECTION('ref_axis',(0.,0.,-1.)) ;
#62948=DIRECTION('center_axis',(0.,1.,7.10542735760115E-13)) ;
#62949=DIRECTION('ref_axis',(-1.,0.,0.)) ;
#62950=DIRECTION('center_axis',(1.,0.,2.52374105052742E-18)) ;
#62951=DIRECTION('ref_axis',(2.40003400727798E-18,-0.309244171891167,-0.950982671845994)) ;
#62952=DIRECTION('',(-1.,0.,-2.52374105052742E-18)) ;
#62953=DIRECTION('',(1.,0.,2.52374105052742E-18)) ;
#62954=DIRECTION('center_axis',(-1.41426179436738E-51,1.,5.60383084497445E-34)) ;
#62955=DIRECTION('ref_axis',(-0.707106781186548,3.96250679110377E-34,-0.707106781186548)) ;
#62956=DIRECTION('',(1.41426179436738E-51,-1.,-5.60383084497445E-34)) ;
#62957=DIRECTION('',(-1.41426179436738E-51,1.,5.60383084497445E-34)) ;
#62958=DIRECTION('center_axis',(0.,0.,1.)) ;
#62959=DIRECTION('ref_axis',(1.,0.,0.)) ;
#62960=DIRECTION('center_axis',(-2.52374105052742E-18,-5.60383084497445E-34,
1.)) ;
#62961=DIRECTION('ref_axis',(-0.707106781186579,0.707106781186516,-1.78455441078688E-18)) ;
#62962=DIRECTION('center_axis',(0.,-1.,0.)) ;
#62963=DIRECTION('ref_axis',(1.,0.,0.)) ;
#62964=DIRECTION('center_axis',(0.,0.,-1.)) ;
#62965=DIRECTION('ref_axis',(0.,1.,0.)) ;
#62966=DIRECTION('center_axis',(1.,0.,0.)) ;
#62967=DIRECTION('ref_axis',(0.,0.,1.)) ;
#62968=DIRECTION('center_axis',(-2.52374105052742E-18,-5.60383084497445E-34,
1.)) ;
#62969=DIRECTION('ref_axis',(1.53047287779293E-16,-1.,-1.7413136165696E-34)) ;
#62970=DIRECTION('center_axis',(1.,0.,0.)) ;
#62971=DIRECTION('ref_axis',(0.,0.588171697675131,0.808736084303127)) ;
#62972=DIRECTION('center_axis',(0.,-0.276379946678561,-0.961048450950292)) ;
#62973=DIRECTION('ref_axis',(0.,-0.961048450950292,0.276379946678561)) ;
#62974=DIRECTION('center_axis',(0.,1.,0.)) ;
#62975=DIRECTION('ref_axis',(0.,0.,1.)) ;
#62976=DIRECTION('center_axis',(-1.41426179436738E-51,1.,5.60383084497445E-34)) ;
#62977=DIRECTION('ref_axis',(0.707106781186485,-3.96250679110413E-34,0.70710678118661)) ;
#62978=DIRECTION('',(1.41426179436738E-51,-1.,-5.60383084497445E-34)) ;
#62979=DIRECTION('',(-1.41426179436738E-51,1.,5.60383084497445E-34)) ;
#62980=DIRECTION('center_axis',(1.,0.,2.52374105052742E-18)) ;
#62981=DIRECTION('ref_axis',(-2.40003400727851E-18,0.309244171890519,0.950982671846205)) ;
#62982=DIRECTION('',(-1.,0.,-2.52374105052742E-18)) ;
#62983=DIRECTION('',(1.,0.,2.52374105052742E-18)) ;
#62984=DIRECTION('center_axis',(1.14376454575628E-51,-0.80873608430319,
0.588171697675045)) ;
#62985=DIRECTION('ref_axis',(-0.707106781186659,-0.415900195927963,-0.571862769400951)) ;
#62986=DIRECTION('',(-1.14376454575628E-51,0.80873608430319,-0.588171697675045)) ;
#62987=DIRECTION('',(1.14376454575628E-51,-0.80873608430319,0.588171697675045)) ;
#62988=DIRECTION('center_axis',(0.,0.,1.)) ;
#62989=DIRECTION('ref_axis',(-0.707106781186862,0.707106781186234,0.)) ;
#62990=DIRECTION('',(0.,0.,-1.)) ;
#62991=DIRECTION('',(0.,0.,1.)) ;
#62992=DIRECTION('center_axis',(1.,0.,2.52374105052742E-18)) ;
#62993=DIRECTION('ref_axis',(-1.78455441078775E-18,-0.707106781186171,0.707106781186924)) ;
#62994=DIRECTION('',(-1.,0.,-2.52374105052742E-18)) ;
#62995=DIRECTION('',(1.,0.,2.52374105052742E-18)) ;
#62996=DIRECTION('center_axis',(0.,0.,1.)) ;
#62997=DIRECTION('ref_axis',(0.707106781186799,0.707106781186296,0.)) ;
#62998=DIRECTION('',(0.,0.,-1.)) ;
#62999=DIRECTION('',(0.,0.,1.)) ;
#63000=DIRECTION('center_axis',(2.52374105052742E-18,5.60383084497445E-34,
-1.)) ;
#63001=DIRECTION('ref_axis',(1.,3.40207761657885E-68,2.52374105052742E-18)) ;
#63002=DIRECTION('center_axis',(0.,1.,0.)) ;
#63003=DIRECTION('ref_axis',(-1.,0.,-2.52374105052742E-18)) ;
#63004=DIRECTION('center_axis',(1.,1.41426179436738E-51,0.)) ;
#63005=DIRECTION('ref_axis',(-1.41426179436738E-51,1.,5.60383084497445E-34)) ;
#63006=DIRECTION('center_axis',(-2.04104045499877E-18,0.588171697675045,
0.80873608430319)) ;
#63007=DIRECTION('ref_axis',(1.,3.0425809505486E-33,2.52374105052742E-18)) ;
#63008=DIRECTION('center_axis',(-1.,-1.41426179436738E-51,0.)) ;
#63009=DIRECTION('ref_axis',(1.41426179436738E-51,-1.,-5.60383084497445E-34)) ;
#63010=DIRECTION('center_axis',(-0.408248290463887,0.408248290463603,-0.816496580927844)) ;
#63011=DIRECTION('ref_axis',(-0.577350269189626,0.577350269189768,0.577350269189484)) ;
#63012=DIRECTION('center_axis',(0.,0.,1.)) ;
#63013=DIRECTION('ref_axis',(-1.,0.,0.)) ;
#63014=DIRECTION('center_axis',(0.,1.,0.)) ;
#63015=DIRECTION('ref_axis',(0.,0.,1.)) ;
#63016=DIRECTION('center_axis',(-1.,0.,8.88178419700144E-14)) ;
#63017=DIRECTION('ref_axis',(0.,1.,0.)) ;
#63018=DIRECTION('center_axis',(0.408248290463875,-0.81649658092775,0.408248290463804)) ;
#63019=DIRECTION('ref_axis',(0.577350269189578,0.577350269189721,0.577350269189578)) ;
#63020=DIRECTION('center_axis',(0.,0.,1.)) ;
#63021=DIRECTION('ref_axis',(0.,1.,0.)) ;
#63022=DIRECTION('center_axis',(1.,0.,0.)) ;
#63023=DIRECTION('ref_axis',(0.,0.,1.)) ;
#63024=DIRECTION('center_axis',(0.,1.,0.)) ;
#63025=DIRECTION('ref_axis',(1.,0.,0.)) ;
#63026=DIRECTION('center_axis',(1.,0.,2.52374105052742E-18)) ;
#63027=DIRECTION('ref_axis',(-1.78455441078759E-18,0.707106781186234,0.707106781186862)) ;
#63028=DIRECTION('',(-1.,0.,-2.52374105052742E-18)) ;
#63029=DIRECTION('',(1.,0.,2.52374105052742E-18)) ;
#63030=DIRECTION('center_axis',(-1.41426179436738E-51,1.,5.60383084497445E-34)) ;
#63031=DIRECTION('ref_axis',(-0.70710678118661,-3.96250679110342E-34,0.707106781186485)) ;
#63032=DIRECTION('',(-1.41426179436738E-51,1.,5.60383084497445E-34)) ;
#63033=DIRECTION('',(1.41426179436738E-51,-1.,-5.60383084497445E-34)) ;
#63034=DIRECTION('center_axis',(-0.707106781186453,0.707106781186642,0.)) ;
#63035=DIRECTION('ref_axis',(-0.707106781186642,-0.707106781186453,-7.92501358220861E-34)) ;
#63036=DIRECTION('center_axis',(0.113208280231592,-0.0586760459202665,-0.991837187708834)) ;
#63037=DIRECTION('ref_axis',(0.880585961402273,-0.456409214963279,0.127510756714242)) ;
#63038=DIRECTION('center_axis',(0.,-0.855197831554128,0.518301716093163)) ;
#63039=DIRECTION('ref_axis',(1.,0.,0.)) ;
#63040=DIRECTION('center_axis',(-7.10542735760115E-13,-1.,0.)) ;
#63041=DIRECTION('ref_axis',(0.,0.,1.)) ;
#63042=DIRECTION('center_axis',(1.,0.,0.)) ;
#63043=DIRECTION('ref_axis',(0.,-0.518301716093565,-0.855197831553884)) ;
#63044=DIRECTION('center_axis',(1.41426179436738E-51,-1.,-5.60383084497445E-34)) ;
#63045=DIRECTION('ref_axis',(0.707106781186485,-3.96250679110413E-34,0.70710678118661)) ;
#63046=DIRECTION('',(-1.41426179436738E-51,1.,5.60383084497445E-34)) ;
#63047=DIRECTION('',(1.41426179436738E-51,-1.,-5.60383084497445E-34)) ;
#63048=DIRECTION('center_axis',(-1.,4.16417273337025E-18,-2.52374105052742E-18)) ;
#63049=DIRECTION('ref_axis',(-4.68966975891094E-18,-0.963119367356714,0.269074495674346)) ;
#63050=DIRECTION('',(1.,-4.16417273337025E-18,2.52374105052742E-18)) ;
#63051=DIRECTION('',(-1.,4.16417273337025E-18,-2.52374105052742E-18)) ;
#63052=DIRECTION('center_axis',(1.,1.41426179436738E-51,0.)) ;
#63053=DIRECTION('ref_axis',(1.36210292466788E-51,-0.963119367356714,0.269074495674346)) ;
#63054=DIRECTION('center_axis',(1.20947361979268E-51,-0.855197831554018,
0.518301716093344)) ;
#63055=DIRECTION('ref_axis',(0.707106781186597,-0.366494658150203,-0.604716185947835)) ;
#63056=DIRECTION('center_axis',(0.,0.,1.)) ;
#63057=DIRECTION('ref_axis',(0.,-1.,0.)) ;
#63058=DIRECTION('',(1.20947361979268E-51,-0.855197831554018,0.518301716093344)) ;
#63059=DIRECTION('',(-1.20947361979268E-51,0.855197831554018,-0.518301716093344)) ;
#63060=DIRECTION('center_axis',(0.,0.,-1.)) ;
#63061=DIRECTION('ref_axis',(0.707106781186799,0.707106781186296,0.)) ;
#63062=DIRECTION('center_axis',(0.,0.,1.)) ;
#63063=DIRECTION('ref_axis',(0.707106781186799,0.707106781186296,0.)) ;
#63064=DIRECTION('',(0.,0.,1.)) ;
#63065=DIRECTION('',(0.,0.,-1.)) ;
#63066=DIRECTION('center_axis',(0.,0.,-1.)) ;
#63067=DIRECTION('ref_axis',(-0.707106781186862,0.707106781186234,0.)) ;
#63068=DIRECTION('center_axis',(0.,0.,1.)) ;
#63069=DIRECTION('ref_axis',(-0.707106781186862,0.707106781186234,0.)) ;
#63070=DIRECTION('',(0.,0.,1.)) ;
#63071=DIRECTION('',(0.,0.,-1.)) ;
#63072=DIRECTION('center_axis',(1.,1.41426179436738E-51,0.)) ;
#63073=DIRECTION('ref_axis',(1.41426179436738E-51,-1.,-5.60383084497445E-34)) ;
#63074=DIRECTION('',(1.41426179436738E-51,-1.,-5.60383084497445E-34)) ;
#63075=DIRECTION('center_axis',(0.,0.,-1.)) ;
#63076=DIRECTION('ref_axis',(-1.,0.,0.)) ;
#63077=DIRECTION('',(1.,0.,0.)) ;
#63078=DIRECTION('',(-1.41426179436738E-51,1.,5.60383084497445E-34)) ;
#63079=DIRECTION('',(1.,0.,2.52374105052742E-18)) ;
#63080=DIRECTION('center_axis',(0.,-0.518301716093344,-0.855197831554018)) ;
#63081=DIRECTION('ref_axis',(-1.,0.,0.)) ;
#63082=DIRECTION('',(-1.20947361979268E-51,0.855197831554018,-0.518301716093344)) ;
#63083=DIRECTION('center_axis',(2.52374105052742E-18,5.60383084497445E-34,
-1.)) ;
#63084=DIRECTION('ref_axis',(1.,3.40207761657885E-68,2.52374105052742E-18)) ;
#63085=DIRECTION('center_axis',(-1.,-1.41426179436738E-51,0.)) ;
#63086=DIRECTION('ref_axis',(-1.41426179436738E-51,1.,5.60383084497445E-34)) ;
#63087=DIRECTION('center_axis',(0.,1.,0.)) ;
#63088=DIRECTION('ref_axis',(1.,0.,2.52374105052742E-18)) ;
#88772=CARTESIAN_POINT('',(0.,0.,0.)) ;
#88773=CARTESIAN_POINT('Origin',(45.05,247.85,28.7713203435596)) ;
#88774=CARTESIAN_POINT('',(45.05,247.9,28.7713203435596)) ;
#88775=CARTESIAN_POINT('',(45.1,247.85,28.7713203435596)) ;
#88776=CARTESIAN_POINT('Origin',(45.05,247.85,28.7713203435596)) ;
#88777=CARTESIAN_POINT('',(45.05,247.85,28.7213203435596)) ;
#88778=CARTESIAN_POINT('Origin',(45.05,247.85,28.7713203435596)) ;
#88779=CARTESIAN_POINT('Origin',(45.05,247.85,28.7713203435596)) ;
#88780=CARTESIAN_POINT('Origin',(45.05,246.91625919068,28.7713203435596)) ;
#88781=CARTESIAN_POINT('',(45.1,246.91625919068,28.7713203435596)) ;
#88782=CARTESIAN_POINT('',(45.05,246.886850605796,28.7308835393444)) ;
#88783=CARTESIAN_POINT('Origin',(45.05,246.91625919068,28.7713203435596)) ;
#88784=CARTESIAN_POINT('',(45.05,246.91625919068,28.7213203435596)) ;
#88785=CARTESIAN_POINT('Origin',(45.05,246.91625919068,28.7713203435596)) ;
#88786=CARTESIAN_POINT('Origin',(45.05,246.91625919068,28.7713203435596)) ;
#88787=CARTESIAN_POINT('Origin',(45.05,247.15,28.7713203435596)) ;
#88788=CARTESIAN_POINT('',(45.1,247.15,28.7713203435596)) ;
#88789=CARTESIAN_POINT('',(45.05,247.15,28.7213203435596)) ;
#88790=CARTESIAN_POINT('Origin',(35.35,247.85,28.7713203435596)) ;
#88791=CARTESIAN_POINT('',(35.35,247.85,28.7213203435596)) ;
#88792=CARTESIAN_POINT('',(35.3,247.85,28.7713203435596)) ;
#88793=CARTESIAN_POINT('Origin',(35.35,247.85,28.7713203435596)) ;
#88794=CARTESIAN_POINT('',(35.35,247.9,28.7713203435596)) ;
#88795=CARTESIAN_POINT('Origin',(35.35,247.85,28.7713203435596)) ;
#88796=CARTESIAN_POINT('Origin',(35.35,247.85,28.7713203435596)) ;
#88797=CARTESIAN_POINT('Origin',(42.65,247.85,28.7713203435596)) ;
#88798=CARTESIAN_POINT('',(42.65,247.9,28.7713203435596)) ;
#88799=CARTESIAN_POINT('',(42.65,247.85,28.7213203435596)) ;
#88800=CARTESIAN_POINT('Origin',(45.05,247.85,31.8713203435596)) ;
#88801=CARTESIAN_POINT('',(45.1,247.85,31.8713203435596)) ;
#88802=CARTESIAN_POINT('',(45.05,247.9,31.8713203435596)) ;
#88803=CARTESIAN_POINT('Origin',(45.05,247.85,31.8713203435596)) ;
#88804=CARTESIAN_POINT('',(45.15,247.85,31.9213203435596)) ;
#88805=CARTESIAN_POINT('Origin',(45.15,247.85,31.8713203435596)) ;
#88806=CARTESIAN_POINT('',(45.05,247.95,31.9213203435596)) ;
#88807=CARTESIAN_POINT('Origin',(45.05,247.85,31.9213203435596)) ;
#88808=CARTESIAN_POINT('Origin',(45.05,247.95,31.8713203435596)) ;
#88809=CARTESIAN_POINT('Ctrl Pts',(45.100000736089,242.654130216336,31.8710061164266)) ;
#88810=CARTESIAN_POINT('Ctrl Pts',(45.0999925613464,242.62245247665,31.8801399127304)) ;
#88811=CARTESIAN_POINT('Ctrl Pts',(45.093399397134,242.569918655277,31.8953123581957)) ;
#88812=CARTESIAN_POINT('Ctrl Pts',(45.0723245052974,242.522754591895,31.9089495529807)) ;
#88813=CARTESIAN_POINT('Ctrl Pts',(45.0573753277667,242.51316005143,31.9117246086577)) ;
#88814=CARTESIAN_POINT('Ctrl Pts',(45.0498683683397,242.513216942934,31.9117081537903)) ;
#88815=CARTESIAN_POINT('Ctrl Pts',(45.0999007385685,242.654129809016,31.8860569433972)) ;
#88816=CARTESIAN_POINT('Ctrl Pts',(45.1027420250355,242.622491185791,31.8934562217455)) ;
#88817=CARTESIAN_POINT('Ctrl Pts',(45.0988440451183,242.5681700861,31.9044544950197)) ;
#88818=CARTESIAN_POINT('Ctrl Pts',(45.0760540091005,242.518481086614,31.9134709137417)) ;
#88819=CARTESIAN_POINT('Ctrl Pts',(45.0585961298263,242.508297013843,31.9152655724638)) ;
#88820=CARTESIAN_POINT('Ctrl Pts',(45.0498465782584,242.508357399168,31.9152549299434)) ;
#88821=CARTESIAN_POINT('Ctrl Pts',(45.1124458017577,242.654149588799,31.9121185269271)) ;
#88822=CARTESIAN_POINT('Ctrl Pts',(45.1168400062175,242.620824309685,31.9143468692785)) ;
#88823=CARTESIAN_POINT('Ctrl Pts',(45.1124356980016,242.56280158586,31.9172670990625)) ;
#88824=CARTESIAN_POINT('Ctrl Pts',(45.0833001042428,242.509598931222,31.9194845333789)) ;
#88825=CARTESIAN_POINT('Ctrl Pts',(45.0610143823453,242.498676245984,31.9198998020343)) ;
#88826=CARTESIAN_POINT('Ctrl Pts',(45.0498034221959,242.498741010382,31.9198973387953)) ;
#88827=CARTESIAN_POINT('Ctrl Pts',(45.138764565538,242.654190410765,31.9213206201139)) ;
#88828=CARTESIAN_POINT('Ctrl Pts',(45.1401144780131,242.617375310913,31.9212968863911)) ;
#88829=CARTESIAN_POINT('Ctrl Pts',(45.129606976681,242.55548089994,31.9213095444323)) ;
#88830=CARTESIAN_POINT('Ctrl Pts',(45.091319078717,242.499569893145,31.9213068206852)) ;
#88831=CARTESIAN_POINT('Ctrl Pts',(45.0636555557442,242.488165179893,31.9213204231679)) ;
#88832=CARTESIAN_POINT('Ctrl Pts',(45.0497562823574,242.488232804192,31.9213203428565)) ;
#88833=CARTESIAN_POINT('Ctrl Pts',(45.1499996370486,242.654207810581,31.9213203435596)) ;
#88834=CARTESIAN_POINT('Ctrl Pts',(45.1500616220573,242.615905236523,31.9213203435596)) ;
#88835=CARTESIAN_POINT('Ctrl Pts',(45.1369492436899,242.552354124405,31.9213203435596)) ;
#88836=CARTESIAN_POINT('Ctrl Pts',(45.094751916561,242.495283622616,31.9213203435596)) ;
#88837=CARTESIAN_POINT('Ctrl Pts',(45.0647843437491,242.483672564324,31.9213203435596)) ;
#88838=CARTESIAN_POINT('Ctrl Pts',(45.049736135378,242.483741412881,31.9213203435596)) ;
#88839=CARTESIAN_POINT('',(45.05,242.48374080932,31.9213203435596)) ;
#88840=CARTESIAN_POINT('',(45.15,242.653759190679,31.9213203435596)) ;
#88841=CARTESIAN_POINT('Origin',(45.05,242.653759190679,31.9213203435596)) ;
#88842=CARTESIAN_POINT('',(45.1,242.653759190679,31.8713203435596)) ;
#88843=CARTESIAN_POINT('Origin',(45.15,242.653759190679,31.8713203435596)) ;
#88844=CARTESIAN_POINT('',(45.05,242.513149394204,31.9117571477748)) ;
#88845=CARTESIAN_POINT('Origin',(45.05,242.653759190679,31.8713203435596)) ;
#88846=CARTESIAN_POINT('Origin',(45.05,242.48374080932,31.8713203435596)) ;
#88847=CARTESIAN_POINT('Origin',(45.15,246.025,31.8713203435596)) ;
#88848=CARTESIAN_POINT('',(45.15,246.025,31.9213203435596)) ;
#88849=CARTESIAN_POINT('',(45.1,246.025,31.8713203435596)) ;
#88850=CARTESIAN_POINT('Origin',(45.05,245.187246422722,30.0287841748018)) ;
#88851=CARTESIAN_POINT('',(45.05,245.157837837838,29.9883473705867)) ;
#88852=CARTESIAN_POINT('',(45.1,245.187246422722,30.0287841748018)) ;
#88853=CARTESIAN_POINT('Origin',(35.35,246.91625919068,28.7713203435596)) ;
#88854=CARTESIAN_POINT('',(35.35,246.886850605796,28.7308835393445)) ;
#88855=CARTESIAN_POINT('',(35.3,246.91625919068,28.7713203435596)) ;
#88856=CARTESIAN_POINT('Origin',(35.35,246.91625919068,28.7713203435596)) ;
#88857=CARTESIAN_POINT('',(35.35,246.91625919068,28.7213203435596)) ;
#88858=CARTESIAN_POINT('Origin',(35.35,246.91625919068,28.7713203435596)) ;
#88859=CARTESIAN_POINT('Origin',(35.35,246.91625919068,28.7713203435596)) ;
#88860=CARTESIAN_POINT('Origin',(38.975,246.91625919068,28.7713203435596)) ;
#88861=CARTESIAN_POINT('',(38.975,246.91625919068,28.7213203435596)) ;
#88862=CARTESIAN_POINT('',(38.975,246.886850605796,28.7308835393445)) ;
#88863=CARTESIAN_POINT('Origin',(35.35,247.65,28.7713203435596)) ;
#88864=CARTESIAN_POINT('',(35.3,247.65,28.7713203435596)) ;
#88865=CARTESIAN_POINT('',(35.35,247.65,28.7213203435596)) ;
#88866=CARTESIAN_POINT('Origin',(35.35,247.85,31.8713203435596)) ;
#88867=CARTESIAN_POINT('',(35.35,247.95,31.9213203435596)) ;
#88868=CARTESIAN_POINT('',(35.25,247.85,31.9213203435596)) ;
#88869=CARTESIAN_POINT('Origin',(35.35,247.85,31.9213203435596)) ;
#88870=CARTESIAN_POINT('',(35.3,247.85,31.8713203435596)) ;
#88871=CARTESIAN_POINT('Origin',(35.25,247.85,31.8713203435596)) ;
#88872=CARTESIAN_POINT('',(35.35,247.9,31.8713203435596)) ;
#88873=CARTESIAN_POINT('Origin',(35.35,247.85,31.8713203435596)) ;
#88874=CARTESIAN_POINT('Origin',(35.35,247.95,31.8713203435596)) ;
#88875=CARTESIAN_POINT('Ctrl Pts',(35.3502565731995,242.513282235284,31.9116610526359)) ;
#88876=CARTESIAN_POINT('Ctrl Pts',(35.3390013657597,242.513112238919,31.9117105145564)) ;
#88877=CARTESIAN_POINT('Ctrl Pts',(35.3126883604354,242.538810184974,31.9042333955065)) ;
#88878=CARTESIAN_POINT('Ctrl Pts',(35.3000170639085,242.612165533139,31.8829377134629)) ;
#88879=CARTESIAN_POINT('Ctrl Pts',(35.299997199836,242.654484026663,31.8707059635828)) ;
#88880=CARTESIAN_POINT('Ctrl Pts',(35.3502992712021,242.508407184294,31.9152313508883)) ;
#88881=CARTESIAN_POINT('Ctrl Pts',(35.3371713310074,242.508226354371,31.9152624722717)) ;
#88882=CARTESIAN_POINT('Ctrl Pts',(35.3063767609757,242.535564204124,31.9105601570622)) ;
#88883=CARTESIAN_POINT('Ctrl Pts',(35.2963540554806,242.612239454015,31.8957701050313)) ;
#88884=CARTESIAN_POINT('Ctrl Pts',(35.3001940210199,242.654482933999,31.8858430843487)) ;
#88885=CARTESIAN_POINT('Ctrl Pts',(35.3503840040175,242.498741118317,31.9199072049728)) ;
#88886=CARTESIAN_POINT('Ctrl Pts',(35.3335389864695,242.498547467106,31.9199143760934)) ;
#88887=CARTESIAN_POINT('Ctrl Pts',(35.2940728826173,242.527823493039,31.9188313538683)) ;
#88888=CARTESIAN_POINT('Ctrl Pts',(35.2816723512703,242.610023632475,31.9151151694671)) ;
#88889=CARTESIAN_POINT('Ctrl Pts',(35.287633530646,242.654521639855,31.9121464449948)) ;
#88890=CARTESIAN_POINT('Ctrl Pts',(35.3504766155513,242.488173521915,31.921328574714)) ;
#88891=CARTESIAN_POINT('Ctrl Pts',(35.3295687857424,242.487971244137,31.9213286024899)) ;
#88892=CARTESIAN_POINT('Ctrl Pts',(35.2806653372481,242.518549809002,31.9213243830799)) ;
#88893=CARTESIAN_POINT('Ctrl Pts',(35.2592374640768,242.605399085081,31.9213249653989)) ;
#88894=CARTESIAN_POINT('Ctrl Pts',(35.2610978069887,242.654602031267,31.9213742951207)) ;
#88895=CARTESIAN_POINT('Ctrl Pts',(35.3505162409945,242.483651681807,31.921320259465)) ;
#88896=CARTESIAN_POINT('Ctrl Pts',(35.3278700899377,242.483445705528,31.9213202584698)) ;
#88897=CARTESIAN_POINT('Ctrl Pts',(35.2749216409559,242.514582707583,31.92132040927)) ;
#88898=CARTESIAN_POINT('Ctrl Pts',(35.2496412591386,242.603428347186,31.9213206187124)) ;
#88899=CARTESIAN_POINT('Ctrl Pts',(35.2497723113216,242.654636290699,31.921319786846)) ;
#88900=CARTESIAN_POINT('',(35.25,242.653759190679,31.9213203435596)) ;
#88901=CARTESIAN_POINT('',(35.35,242.48374080932,31.9213203435596)) ;
#88902=CARTESIAN_POINT('Origin',(35.35,242.65375919068,31.9213203435596)) ;
#88903=CARTESIAN_POINT('',(35.35,242.513149394204,31.9117571477748)) ;
#88904=CARTESIAN_POINT('Origin',(35.35,242.48374080932,31.8713203435596)) ;
#88905=CARTESIAN_POINT('',(35.3,242.653759190679,31.8713203435596)) ;
#88906=CARTESIAN_POINT('Origin',(35.35,242.65375919068,31.8713203435596)) ;
#88907=CARTESIAN_POINT('Origin',(35.25,242.653759190679,31.8713203435596)) ;
#88908=CARTESIAN_POINT('Origin',(35.25,246.525,31.8713203435596)) ;
#88909=CARTESIAN_POINT('',(35.25,246.525,31.9213203435596)) ;
#88910=CARTESIAN_POINT('',(35.3,246.525,31.8713203435596)) ;
#88911=CARTESIAN_POINT('Origin',(38.975,242.48374080932,31.8713203435596)) ;
#88912=CARTESIAN_POINT('',(38.975,242.513149394204,31.9117571477748)) ;
#88913=CARTESIAN_POINT('',(38.975,242.48374080932,31.9213203435596)) ;
#88914=CARTESIAN_POINT('Origin',(35.35,245.514273449749,29.790946336964)) ;
#88915=CARTESIAN_POINT('',(35.35,245.484864864865,29.7505095327488)) ;
#88916=CARTESIAN_POINT('',(35.3,245.514273449749,29.790946336964)) ;
#88917=CARTESIAN_POINT('Origin',(35.35,247.85,31.4213203435596)) ;
#88918=CARTESIAN_POINT('',(35.3,247.85,31.4213203435596)) ;
#88919=CARTESIAN_POINT('',(35.35,247.9,31.4213203435596)) ;
#88920=CARTESIAN_POINT('Origin',(42.65,247.95,31.8713203435596)) ;
#88921=CARTESIAN_POINT('',(42.65,247.95,31.9213203435596)) ;
#88922=CARTESIAN_POINT('',(42.65,247.9,31.8713203435596)) ;
#88923=CARTESIAN_POINT('Origin',(45.05,247.85,31.4213203435596)) ;
#88924=CARTESIAN_POINT('',(45.05,247.9,31.4213203435596)) ;
#88925=CARTESIAN_POINT('',(45.1,247.85,31.4213203435596)) ;
#88926=CARTESIAN_POINT('Origin',(40.2,247.4,28.7213203435596)) ;
#88927=CARTESIAN_POINT('Origin',(45.1,247.9,31.4213203435596)) ;
#88928=CARTESIAN_POINT('Origin',(45.1,246.9,31.4213203435596)) ;
#88929=CARTESIAN_POINT('Origin',(37.75,244.7,30.3213203435596)) ;
#88930=CARTESIAN_POINT('Origin',(35.3,247.9,31.4213203435596)) ;
#88931=CARTESIAN_POINT('Origin',(34.35,248.85,31.8713203435596)) ;
#88932=CARTESIAN_POINT('',(34.3,248.85,31.8713203435596)) ;
#88933=CARTESIAN_POINT('',(34.35,248.9,31.8713203435596)) ;
#88934=CARTESIAN_POINT('Origin',(34.35,248.85,31.8713203435596)) ;
#88935=CARTESIAN_POINT('',(34.35,248.85,31.9213203435596)) ;
#88936=CARTESIAN_POINT('Origin',(34.35,248.85,31.8713203435596)) ;
#88937=CARTESIAN_POINT('Origin',(34.35,248.85,31.8713203435596)) ;
#88938=CARTESIAN_POINT('Origin',(46.05,248.85,31.8713203435596)) ;
#88939=CARTESIAN_POINT('',(46.05,248.9,31.8713203435596)) ;
#88940=CARTESIAN_POINT('',(46.1,248.85,31.8713203435596)) ;
#88941=CARTESIAN_POINT('Origin',(46.05,248.85,31.8713203435596)) ;
#88942=CARTESIAN_POINT('',(46.05,248.85,31.9213203435596)) ;
#88943=CARTESIAN_POINT('Origin',(46.05,248.85,31.8713203435596)) ;
#88944=CARTESIAN_POINT('Origin',(46.05,248.85,31.8713203435596)) ;
#88945=CARTESIAN_POINT('Origin',(37.25,248.85,31.8713203435596)) ;
#88946=CARTESIAN_POINT('',(37.25,248.9,31.8713203435596)) ;
#88947=CARTESIAN_POINT('',(37.25,248.85,31.9213203435596)) ;
#88948=CARTESIAN_POINT('Origin',(34.35,243.275,31.8713203435596)) ;
#88949=CARTESIAN_POINT('',(34.35,241.578968906908,31.9213203435596)) ;
#88950=CARTESIAN_POINT('',(34.35,243.275,31.9213203435596)) ;
#88951=CARTESIAN_POINT('',(34.3,241.528968906908,31.8713203435596)) ;
#88952=CARTESIAN_POINT('',(34.3,243.275,31.8713203435596)) ;
#88953=CARTESIAN_POINT('Origin',(34.35,241.578968906908,31.8713203435596)) ;
#88954=CARTESIAN_POINT('Origin',(46.05,241.578968906908,31.8713203435596)) ;
#88955=CARTESIAN_POINT('',(46.1,241.578968906908,31.8713203435596)) ;
#88956=CARTESIAN_POINT('',(46.05,241.553053821103,31.8285604519819)) ;
#88957=CARTESIAN_POINT('Origin',(46.05,241.578968906908,31.8713203435596)) ;
#88958=CARTESIAN_POINT('',(46.05,241.578968906908,31.9213203435596)) ;
#88959=CARTESIAN_POINT('Origin',(46.05,241.578968906908,31.8713203435596)) ;
#88960=CARTESIAN_POINT('Origin',(46.05,241.578968906908,31.8713203435596)) ;
#88961=CARTESIAN_POINT('Origin',(46.05,247.025,31.8713203435596)) ;
#88962=CARTESIAN_POINT('',(46.1,247.025,31.8713203435596)) ;
#88963=CARTESIAN_POINT('',(46.05,247.025,31.9213203435596)) ;
#88964=CARTESIAN_POINT('Origin',(41.675,241.578968906908,31.8713203435596)) ;
#88965=CARTESIAN_POINT('',(34.3,241.553053821103,31.8285604519819)) ;
#88966=CARTESIAN_POINT('',(41.675,241.553053821103,31.8285604519819)) ;
#88967=CARTESIAN_POINT('',(41.675,241.578968906908,31.9213203435596)) ;
#88968=CARTESIAN_POINT('Origin',(34.3,241.578968906908,31.8713203435596)) ;
#88969=CARTESIAN_POINT('Origin',(46.05,245.81852757741,29.3018908462858)) ;
#88970=CARTESIAN_POINT('',(46.05,248.,27.9213203435596)) ;
#88971=CARTESIAN_POINT('',(46.1,248.096468906908,27.9213203435596)) ;
#88972=CARTESIAN_POINT('Origin',(46.05,248.096468906908,27.9213203435596)) ;
#88973=CARTESIAN_POINT('',(46.1,245.81852757741,29.3018908462858)) ;
#88974=CARTESIAN_POINT('',(46.05,245.792612491605,29.2591309547081)) ;
#88975=CARTESIAN_POINT('Origin',(46.05,248.85,31.9213203435596)) ;
#88976=CARTESIAN_POINT('',(46.1,248.85,27.9213203435596)) ;
#88977=CARTESIAN_POINT('',(46.05,248.9,27.9213203435596)) ;
#88978=CARTESIAN_POINT('Origin',(46.05,248.85,27.9213203435596)) ;
#88979=CARTESIAN_POINT('',(46.05,248.9,31.9213203435596)) ;
#88980=CARTESIAN_POINT('',(46.1,248.85,31.9213203435596)) ;
#88981=CARTESIAN_POINT('Origin',(34.35,248.85,31.9213203435596)) ;
#88982=CARTESIAN_POINT('',(34.35,248.9,27.9213203435596)) ;
#88983=CARTESIAN_POINT('',(34.3,248.85,27.9213203435596)) ;
#88984=CARTESIAN_POINT('Origin',(34.35,248.85,27.9213203435596)) ;
#88985=CARTESIAN_POINT('',(34.3,248.85,31.9213203435596)) ;
#88986=CARTESIAN_POINT('',(34.35,248.9,31.9213203435596)) ;
#88987=CARTESIAN_POINT('Origin',(46.1,248.9,31.9213203435596)) ;
#88988=CARTESIAN_POINT('',(46.1,248.9,27.9213203435596)) ;
#88989=CARTESIAN_POINT('Origin',(40.2,245.15,27.9213203435596)) ;
#88990=CARTESIAN_POINT('',(34.3,248.,27.9213203435596)) ;
#88991=CARTESIAN_POINT('',(43.15,248.,27.9213203435596)) ;
#88992=CARTESIAN_POINT('',(34.3,241.4,27.9213203435596)) ;
#88993=CARTESIAN_POINT('',(34.3,248.9,27.9213203435596)) ;
#88994=CARTESIAN_POINT('Origin',(43.15,244.7,29.9213203435596)) ;
#88995=CARTESIAN_POINT('',(34.3,243.05,30.9213203435596)) ;
#88996=CARTESIAN_POINT('Origin',(40.2,245.15,31.9213203435596)) ;
#88997=CARTESIAN_POINT('Origin',(34.3,241.4,31.9213203435596)) ;
#88998=CARTESIAN_POINT('Origin',(34.3,248.9,31.9213203435596)) ;
#117140=UNCERTAINTY_MEASURE_WITH_UNIT(LENGTH_MEASURE(0.01),#117171,
'DISTANCE_ACCURACY_VALUE',
'Maximum model space distance between geometric entities at asserted c
onnectivities') ;
#117147=UNCERTAINTY_MEASURE_WITH_UNIT(LENGTH_MEASURE(0.01),#117171,
'DISTANCE_ACCURACY_VALUE',
'Maximum model space distance between geometric entities at asserted c
onnectivities') ;
#117163=(
GEOMETRIC_REPRESENTATION_CONTEXT(3)
GLOBAL_UNCERTAINTY_ASSIGNED_CONTEXT((#117140))
GLOBAL_UNIT_ASSIGNED_CONTEXT((#117171,#117173,#117174))
REPRESENTATION_CONTEXT('','3D')
) ;
#117170=(
GEOMETRIC_REPRESENTATION_CONTEXT(3)
GLOBAL_UNCERTAINTY_ASSIGNED_CONTEXT((#117147))
GLOBAL_UNIT_ASSIGNED_CONTEXT((#117171,#117173,#117174))
REPRESENTATION_CONTEXT('','3D')
) ;
#117171=(
LENGTH_UNIT()
NAMED_UNIT(*)
SI_UNIT(.MILLI.,.METRE.)
) ;
#117173=(
NAMED_UNIT(*)
PLANE_ANGLE_UNIT()
SI_UNIT($,.RADIAN.)
) ;
#117174=(
NAMED_UNIT(*)
SI_UNIT($,.STERADIAN.)
SOLID_ANGLE_UNIT()
) ;
#117190=SHAPE_DEFINITION_REPRESENTATION(#117212,#117255) ;
#117212=PRODUCT_DEFINITION_SHAPE('',$,#117278) ;
#117255=SHAPE_REPRESENTATION('',(#52444),#117163) ;
#117262=PRODUCT_DEFINITION_CONTEXT('part definition',#117330,'design') ;
#117278=PRODUCT_DEFINITION('Latch','Latch',#117300,#117262) ;
#117300=PRODUCT_DEFINITION_FORMATION('',$,#117347) ;
#117330=APPLICATION_CONTEXT(
'Core Data for Automotive Mechanical Design Process') ;
#117331=PRODUCT_CONTEXT('part definition',#117330,'mechanical') ;
#117347=PRODUCT('Latch','Latch',$,(#117331)) ;
#117355=PRESENTATION_STYLE_ASSIGNMENT((#117357)) ;
#117357=SURFACE_STYLE_USAGE(.BOTH.,#117359) ;
#117359=SURFACE_SIDE_STYLE('',(#117361)) ;
#117361=SURFACE_STYLE_FILL_AREA(#117363) ;
#117363=FILL_AREA_STYLE('Opaque(160,160,160)',(#117365)) ;
#117365=FILL_AREA_STYLE_COLOUR('Opaque(160,160,160)',#117367) ;
#117367=COLOUR_RGB('Opaque(160,160,160)', 0.09019608, 0.27058824, 0.51372549) ;
ENDSEC;
END-ISO-10303-21;
